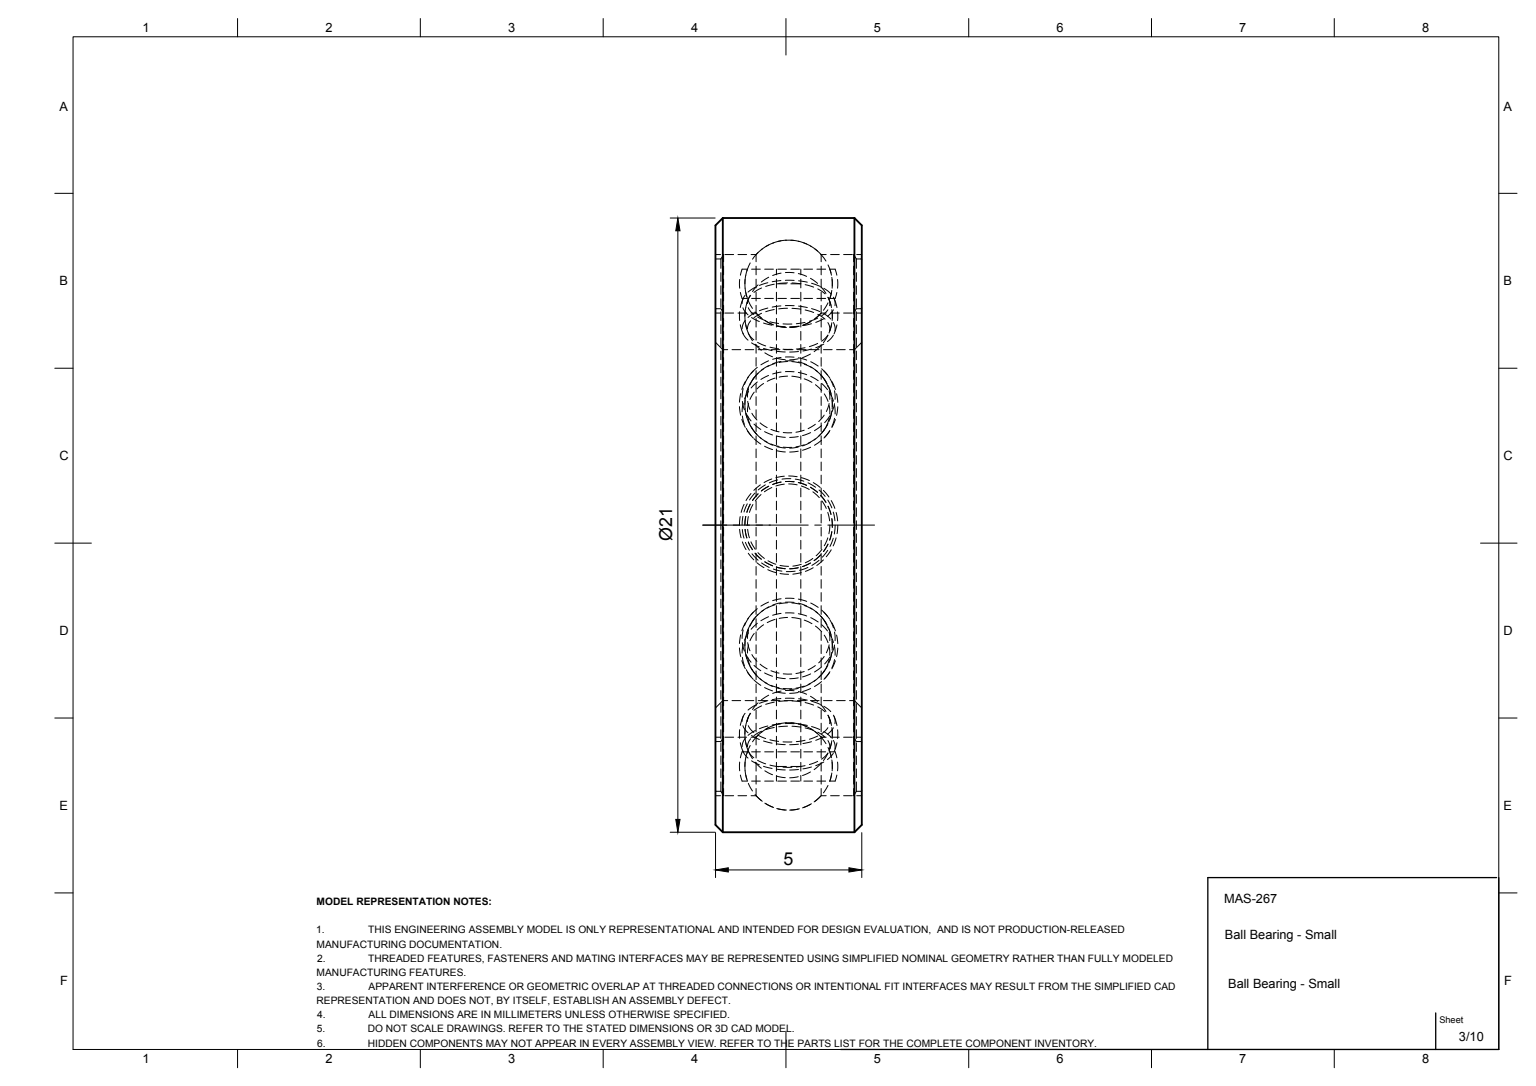
ISO-10303-21;
HEADER;
/* Generated by software containing ST-Developer
 * from STEP Tools, Inc. (www.steptools.com) 
 */

FILE_DESCRIPTION(
/* description */ (''),
/* implementation_level */ '2;1');

FILE_NAME(
/* name */ 'Ball Bearing - Small.step',
/* time_stamp */ '2026-10-12T15:29:24-07:00',
/* author */ (''),
/* organization */ (''),
/* preprocessor_version */ 'ST-DEVELOPER v20.2',
/* originating_system */ 'Autodesk Translation Framework v15.15.0.0',
/* authorisation */ '');

FILE_SCHEMA (('AUTOMOTIVE_DESIGN { 1 0 10303 214 3 1 1 }'));
ENDSEC;

DATA;
#10=MECHANICAL_DESIGN_GEOMETRIC_PRESENTATION_REPRESENTATION('',(#165,#166,#167,#168,#169,#170,#171,#172,#173,#174,#175,#176,#177,#178,#179,#180,#181,#182,#183,#184,#185,#186,#187,#188,#189,#190,#191,#192,#193),#9496);
#95=(
BOUNDED_SURFACE()
B_SPLINE_SURFACE(2,2,((#7928,#7929,#7930,#7931,#7932,#7933,#7934,#7935,
#7936),(#7937,#7938,#7939,#7940,#7941,#7942,#7943,#7944,#7945),(#7946,#7947,
#7948,#7949,#7950,#7951,#7952,#7953,#7954)),.UNSPECIFIED.,.F.,.T.,.F.)
B_SPLINE_SURFACE_WITH_KNOTS((3,3),(3,2,2,2,3),(-0.359817990374321,0.359817990374321),
(-3.14159265358979,-1.5707963267949,0.,1.5707963267949,3.14159265358979),
 .UNSPECIFIED.)
GEOMETRIC_REPRESENTATION_ITEM()
RATIONAL_B_SPLINE_SURFACE(((1.,0.707106781186548,1.,0.707106781186548,1.,
0.707106781186548,1.,0.707106781186548,1.),(0.935960925476955,0.661824317330392,
0.935960925476955,0.661824317330392,0.935960925476955,0.661824317330392,
0.935960925476955,0.661824317330392,0.935960925476955),(1.,0.707106781186548,
1.,0.707106781186548,1.,0.707106781186548,1.,0.707106781186548,1.)))
REPRESENTATION_ITEM('')
SURFACE()
);
#96=(
BOUNDED_SURFACE()
B_SPLINE_SURFACE(2,2,((#7970,#7971,#7972,#7973,#7974,#7975,#7976,#7977,
#7978),(#7979,#7980,#7981,#7982,#7983,#7984,#7985,#7986,#7987),(#7988,#7989,
#7990,#7991,#7992,#7993,#7994,#7995,#7996)),.UNSPECIFIED.,.F.,.T.,.F.)
B_SPLINE_SURFACE_WITH_KNOTS((3,3),(3,2,2,2,3),(-0.359817990374415,0.359817990374426),
(-3.14159265358979,-1.5707963267949,0.,1.5707963267949,3.14159265358979),
 .UNSPECIFIED.)
GEOMETRIC_REPRESENTATION_ITEM()
RATIONAL_B_SPLINE_SURFACE(((1.,0.707106781186548,1.,0.707106781186548,1.,
0.707106781186548,1.,0.707106781186548,1.),(0.935960925476919,0.661824317330366,
0.935960925476919,0.661824317330366,0.935960925476919,0.661824317330366,
0.935960925476919,0.661824317330366,0.935960925476919),(1.,0.707106781186548,
1.,0.707106781186548,1.,0.707106781186548,1.,0.707106781186548,1.)))
REPRESENTATION_ITEM('')
SURFACE()
);
#97=(
BOUNDED_SURFACE()
B_SPLINE_SURFACE(2,2,((#8012,#8013,#8014,#8015,#8016,#8017,#8018,#8019,
#8020),(#8021,#8022,#8023,#8024,#8025,#8026,#8027,#8028,#8029),(#8030,#8031,
#8032,#8033,#8034,#8035,#8036,#8037,#8038)),.UNSPECIFIED.,.F.,.T.,.F.)
B_SPLINE_SURFACE_WITH_KNOTS((3,3),(3,2,2,2,3),(-0.359817990374342,0.359817990374333),
(-3.14159265358979,-1.5707963267949,0.,1.5707963267949,3.14159265358979),
 .UNSPECIFIED.)
GEOMETRIC_REPRESENTATION_ITEM()
RATIONAL_B_SPLINE_SURFACE(((1.,0.707106781186548,1.,0.707106781186548,1.,
0.707106781186548,1.,0.707106781186548,1.),(0.935960925476941,0.661824317330382,
0.935960925476941,0.661824317330382,0.935960925476941,0.661824317330382,
0.935960925476941,0.661824317330382,0.935960925476941),(1.,0.707106781186548,
1.,0.707106781186548,1.,0.707106781186548,1.,0.707106781186548,1.)))
REPRESENTATION_ITEM('')
SURFACE()
);
#98=(
BOUNDED_SURFACE()
B_SPLINE_SURFACE(2,2,((#8054,#8055,#8056,#8057,#8058,#8059,#8060,#8061,
#8062),(#8063,#8064,#8065,#8066,#8067,#8068,#8069,#8070,#8071),(#8072,#8073,
#8074,#8075,#8076,#8077,#8078,#8079,#8080)),.UNSPECIFIED.,.F.,.T.,.F.)
B_SPLINE_SURFACE_WITH_KNOTS((3,3),(3,2,2,2,3),(-0.359817990374327,0.359817990374343),
(-3.14159265358979,-1.5707963267949,0.,1.5707963267949,3.14159265358979),
 .UNSPECIFIED.)
GEOMETRIC_REPRESENTATION_ITEM()
RATIONAL_B_SPLINE_SURFACE(((1.,0.707106781186548,1.,0.707106781186548,1.,
0.707106781186548,1.,0.707106781186548,1.),(0.935960925476945,0.661824317330385,
0.935960925476945,0.661824317330385,0.935960925476945,0.661824317330385,
0.935960925476945,0.661824317330385,0.935960925476945),(1.,0.707106781186548,
1.,0.707106781186548,1.,0.707106781186548,1.,0.707106781186548,1.)))
REPRESENTATION_ITEM('')
SURFACE()
);
#99=(
BOUNDED_SURFACE()
B_SPLINE_SURFACE(2,2,((#8096,#8097,#8098,#8099,#8100,#8101,#8102,#8103,
#8104),(#8105,#8106,#8107,#8108,#8109,#8110,#8111,#8112,#8113),(#8114,#8115,
#8116,#8117,#8118,#8119,#8120,#8121,#8122)),.UNSPECIFIED.,.F.,.T.,.F.)
B_SPLINE_SURFACE_WITH_KNOTS((3,3),(3,2,2,2,3),(-0.359817990374369,0.359817990374379),
(-3.14159265358979,-1.5707963267949,0.,1.5707963267949,3.14159265358979),
 .UNSPECIFIED.)
GEOMETRIC_REPRESENTATION_ITEM()
RATIONAL_B_SPLINE_SURFACE(((1.,0.707106781186548,1.,0.707106781186548,1.,
0.707106781186548,1.,0.707106781186548,1.),(0.935960925476939,0.661824317330381,
0.935960925476939,0.661824317330381,0.935960925476939,0.661824317330381,
0.935960925476939,0.661824317330381,0.935960925476939),(1.,0.707106781186548,
1.,0.707106781186548,1.,0.707106781186548,1.,0.707106781186548,1.)))
REPRESENTATION_ITEM('')
SURFACE()
);
#100=(
BOUNDED_SURFACE()
B_SPLINE_SURFACE(2,2,((#8138,#8139,#8140,#8141,#8142,#8143,#8144,#8145,
#8146),(#8147,#8148,#8149,#8150,#8151,#8152,#8153,#8154,#8155),(#8156,#8157,
#8158,#8159,#8160,#8161,#8162,#8163,#8164)),.UNSPECIFIED.,.F.,.T.,.F.)
B_SPLINE_SURFACE_WITH_KNOTS((3,3),(3,2,2,2,3),(-0.359817990374391,0.359817990374391),
(-3.14159265358979,-1.5707963267949,0.,1.5707963267949,3.14159265358979),
 .UNSPECIFIED.)
GEOMETRIC_REPRESENTATION_ITEM()
RATIONAL_B_SPLINE_SURFACE(((1.,0.707106781186548,1.,0.707106781186548,1.,
0.707106781186548,1.,0.707106781186548,1.),(0.935960925476929,0.661824317330373,
0.935960925476929,0.661824317330373,0.935960925476929,0.661824317330373,
0.935960925476929,0.661824317330373,0.935960925476929),(1.,0.707106781186548,
1.,0.707106781186548,1.,0.707106781186548,1.,0.707106781186548,1.)))
REPRESENTATION_ITEM('')
SURFACE()
);
#101=(
BOUNDED_SURFACE()
B_SPLINE_SURFACE(2,2,((#8180,#8181,#8182,#8183,#8184,#8185,#8186,#8187,
#8188),(#8189,#8190,#8191,#8192,#8193,#8194,#8195,#8196,#8197),(#8198,#8199,
#8200,#8201,#8202,#8203,#8204,#8205,#8206)),.UNSPECIFIED.,.F.,.T.,.F.)
B_SPLINE_SURFACE_WITH_KNOTS((3,3),(3,2,2,2,3),(-0.359817990374328,0.359817990374325),
(-3.14159265358979,-1.5707963267949,0.,1.5707963267949,3.14159265358979),
 .UNSPECIFIED.)
GEOMETRIC_REPRESENTATION_ITEM()
RATIONAL_B_SPLINE_SURFACE(((1.,0.707106781186548,1.,0.707106781186548,1.,
0.707106781186548,1.,0.707106781186548,1.),(0.935960925476951,0.661824317330389,
0.935960925476951,0.661824317330389,0.935960925476951,0.661824317330389,
0.935960925476951,0.661824317330389,0.935960925476951),(1.,0.707106781186548,
1.,0.707106781186548,1.,0.707106781186548,1.,0.707106781186548,1.)))
REPRESENTATION_ITEM('')
SURFACE()
);
#102=(
BOUNDED_SURFACE()
B_SPLINE_SURFACE(2,2,((#8222,#8223,#8224,#8225,#8226,#8227,#8228,#8229,
#8230),(#8231,#8232,#8233,#8234,#8235,#8236,#8237,#8238,#8239),(#8240,#8241,
#8242,#8243,#8244,#8245,#8246,#8247,#8248)),.UNSPECIFIED.,.F.,.T.,.F.)
B_SPLINE_SURFACE_WITH_KNOTS((3,3),(3,2,2,2,3),(-0.359817990374346,0.359817990374343),
(-3.14159265358979,-1.5707963267949,0.,1.5707963267949,3.14159265358979),
 .UNSPECIFIED.)
GEOMETRIC_REPRESENTATION_ITEM()
RATIONAL_B_SPLINE_SURFACE(((1.,0.707106781186548,1.,0.707106781186548,1.,
0.707106781186548,1.,0.707106781186548,1.),(0.935960925476942,0.661824317330383,
0.935960925476942,0.661824317330383,0.935960925476942,0.661824317330383,
0.935960925476942,0.661824317330383,0.935960925476942),(1.,0.707106781186548,
1.,0.707106781186548,1.,0.707106781186548,1.,0.707106781186548,1.)))
REPRESENTATION_ITEM('')
SURFACE()
);
#103=(
BOUNDED_SURFACE()
B_SPLINE_SURFACE(2,2,((#8264,#8265,#8266,#8267,#8268,#8269,#8270,#8271,
#8272),(#8273,#8274,#8275,#8276,#8277,#8278,#8279,#8280,#8281),(#8282,#8283,
#8284,#8285,#8286,#8287,#8288,#8289,#8290)),.UNSPECIFIED.,.F.,.T.,.F.)
B_SPLINE_SURFACE_WITH_KNOTS((3,3),(3,2,2,2,3),(-0.359817990374353,0.359817990374347),
(-3.14159265358979,-1.5707963267949,0.,1.5707963267949,3.14159265358979),
 .UNSPECIFIED.)
GEOMETRIC_REPRESENTATION_ITEM()
RATIONAL_B_SPLINE_SURFACE(((1.,0.707106781186548,1.,0.707106781186548,1.,
0.707106781186548,1.,0.707106781186548,1.),(0.935960925476944,0.661824317330384,
0.935960925476944,0.661824317330384,0.935960925476944,0.661824317330384,
0.935960925476944,0.661824317330384,0.935960925476944),(1.,0.707106781186548,
1.,0.707106781186548,1.,0.707106781186548,1.,0.707106781186548,1.)))
REPRESENTATION_ITEM('')
SURFACE()
);
#104=(
BOUNDED_SURFACE()
B_SPLINE_SURFACE(2,2,((#8306,#8307,#8308,#8309,#8310,#8311,#8312,#8313,
#8314),(#8315,#8316,#8317,#8318,#8319,#8320,#8321,#8322,#8323),(#8324,#8325,
#8326,#8327,#8328,#8329,#8330,#8331,#8332)),.UNSPECIFIED.,.F.,.T.,.F.)
B_SPLINE_SURFACE_WITH_KNOTS((3,3),(3,2,2,2,3),(-0.359817990374389,0.359817990374389),
(-3.14159265358979,-1.5707963267949,0.,1.5707963267949,3.14159265358979),
 .UNSPECIFIED.)
GEOMETRIC_REPRESENTATION_ITEM()
RATIONAL_B_SPLINE_SURFACE(((1.,0.707106781186548,1.,0.707106781186548,1.,
0.707106781186548,1.,0.707106781186548,1.),(0.935960925476925,0.661824317330371,
0.935960925476925,0.661824317330371,0.935960925476925,0.661824317330371,
0.935960925476925,0.661824317330371,0.935960925476925),(1.,0.707106781186548,
1.,0.707106781186548,1.,0.707106781186548,1.,0.707106781186548,1.)))
REPRESENTATION_ITEM('')
SURFACE()
);
#105=(
BOUNDED_SURFACE()
B_SPLINE_SURFACE(2,2,((#8362,#8363,#8364,#8365,#8366,#8367,#8368,#8369,
#8370),(#8371,#8372,#8373,#8374,#8375,#8376,#8377,#8378,#8379),(#8380,#8381,
#8382,#8383,#8384,#8385,#8386,#8387,#8388)),.UNSPECIFIED.,.F.,.T.,.F.)
B_SPLINE_SURFACE_WITH_KNOTS((3,3),(3,2,2,2,3),(-0.359817990374337,0.359817990374338),
(-3.14159265358979,-1.5707963267949,0.,1.5707963267949,3.14159265358979),
 .UNSPECIFIED.)
GEOMETRIC_REPRESENTATION_ITEM()
RATIONAL_B_SPLINE_SURFACE(((1.,0.707106781186548,1.,0.707106781186548,1.,
0.707106781186548,1.,0.707106781186548,1.),(0.935960925476947,0.661824317330386,
0.935960925476947,0.661824317330386,0.935960925476947,0.661824317330386,
0.935960925476947,0.661824317330386,0.935960925476947),(1.,0.707106781186548,
1.,0.707106781186548,1.,0.707106781186548,1.,0.707106781186548,1.)))
REPRESENTATION_ITEM('')
SURFACE()
);
#106=(
BOUNDED_SURFACE()
B_SPLINE_SURFACE(2,2,((#8404,#8405,#8406,#8407,#8408,#8409,#8410,#8411,
#8412),(#8413,#8414,#8415,#8416,#8417,#8418,#8419,#8420,#8421),(#8422,#8423,
#8424,#8425,#8426,#8427,#8428,#8429,#8430)),.UNSPECIFIED.,.F.,.T.,.F.)
B_SPLINE_SURFACE_WITH_KNOTS((3,3),(3,2,2,2,3),(-0.359817990374313,0.359817990374317),
(-3.14159265358979,-1.5707963267949,0.,1.5707963267949,3.14159265358979),
 .UNSPECIFIED.)
GEOMETRIC_REPRESENTATION_ITEM()
RATIONAL_B_SPLINE_SURFACE(((1.,0.707106781186548,1.,0.707106781186548,1.,
0.707106781186548,1.,0.707106781186548,1.),(0.935960925476952,0.66182431733039,
0.935960925476952,0.66182431733039,0.935960925476952,0.66182431733039,0.935960925476952,
0.66182431733039,0.935960925476952),(1.,0.707106781186548,1.,0.707106781186548,
1.,0.707106781186548,1.,0.707106781186548,1.)))
REPRESENTATION_ITEM('')
SURFACE()
);
#107=CONICAL_SURFACE('',#5303,6.24999999999999,0.785398163397428);
#108=CONICAL_SURFACE('',#5309,6.,0.785398163397428);
#109=CONICAL_SURFACE('',#5319,10.25,0.785398163397433);
#110=CONICAL_SURFACE('',#5330,10.5,0.785398163397433);
#111=CONICAL_SURFACE('',#5488,9.25000000000001,1.01776488264426);
#112=CONICAL_SURFACE('',#5490,7.39999999999999,1.01776488264426);
#113=CONICAL_SURFACE('',#5507,7.24999999999999,1.01776488264426);
#114=CONICAL_SURFACE('',#5509,9.1,1.01776488264426);
#124=TOROIDAL_SURFACE('',#5299,8.25,1.49484711634153);
#125=TOROIDAL_SURFACE('',#5325,8.25,1.49484711634153);
#126=TOROIDAL_SURFACE('',#5475,7.42777777777777,0.0277777777777778);
#127=TOROIDAL_SURFACE('',#5480,9.07222222222223,0.0277777777777778);
#128=TOROIDAL_SURFACE('',#5496,9.07222222222222,0.027777777777778);
#129=TOROIDAL_SURFACE('',#5500,7.42777777777777,0.027777777777778);
#147=SHAPE_REPRESENTATION_RELATIONSHIP('SRR','None',#9541,#156);
#156=ADVANCED_BREP_SHAPE_REPRESENTATION('',(#222,#223,#224,#225,#226,#227,
#228,#229,#230,#231,#232,#233,#234,#235,#236,#237,#238,#239,#240,#241,#242,
#243,#244,#245,#246,#247,#248,#249,#250),#9489);
#165=STYLED_ITEM('',(#9594),#222);
#166=STYLED_ITEM('',(#9594),#223);
#167=STYLED_ITEM('',(#9594),#224);
#168=STYLED_ITEM('',(#9594),#225);
#169=STYLED_ITEM('',(#9594),#226);
#170=STYLED_ITEM('',(#9594),#227);
#171=STYLED_ITEM('',(#9594),#228);
#172=STYLED_ITEM('',(#9594),#229);
#173=STYLED_ITEM('',(#9594),#230);
#174=STYLED_ITEM('',(#9594),#231);
#175=STYLED_ITEM('',(#9594),#232);
#176=STYLED_ITEM('',(#9594),#233);
#177=STYLED_ITEM('',(#9594),#234);
#178=STYLED_ITEM('',(#9594),#235);
#179=STYLED_ITEM('',(#9594),#236);
#180=STYLED_ITEM('',(#9594),#237);
#181=STYLED_ITEM('',(#9594),#238);
#182=STYLED_ITEM('',(#9594),#239);
#183=STYLED_ITEM('',(#9594),#240);
#184=STYLED_ITEM('',(#9594),#241);
#185=STYLED_ITEM('',(#9594),#242);
#186=STYLED_ITEM('',(#9594),#243);
#187=STYLED_ITEM('',(#9594),#244);
#188=STYLED_ITEM('',(#9594),#245);
#189=STYLED_ITEM('',(#9594),#246);
#190=STYLED_ITEM('',(#9594),#247);
#191=STYLED_ITEM('',(#9594),#248);
#192=STYLED_ITEM('',(#9594),#249);
#193=STYLED_ITEM('',(#9594),#250);
#222=MANIFOLD_SOLID_BREP('Body1',#4967);
#223=MANIFOLD_SOLID_BREP('Body2',#4968);
#224=MANIFOLD_SOLID_BREP('Body3',#4969);
#225=MANIFOLD_SOLID_BREP('Body4',#4970);
#226=MANIFOLD_SOLID_BREP('Body5',#4971);
#227=MANIFOLD_SOLID_BREP('Body6',#4972);
#228=MANIFOLD_SOLID_BREP('Body7',#4973);
#229=MANIFOLD_SOLID_BREP('Body8',#4974);
#230=MANIFOLD_SOLID_BREP('Body9',#4975);
#231=MANIFOLD_SOLID_BREP('Body10',#4976);
#232=MANIFOLD_SOLID_BREP('Body11',#4977);
#233=MANIFOLD_SOLID_BREP('Body12',#4978);
#234=MANIFOLD_SOLID_BREP('Body13',#4979);
#235=MANIFOLD_SOLID_BREP('Body14',#4980);
#236=MANIFOLD_SOLID_BREP('Body15',#4981);
#237=MANIFOLD_SOLID_BREP('Body16',#4982);
#238=MANIFOLD_SOLID_BREP('Body17',#4983);
#239=MANIFOLD_SOLID_BREP('Body18',#4984);
#240=MANIFOLD_SOLID_BREP('Body19',#4985);
#241=MANIFOLD_SOLID_BREP('Body20',#4986);
#242=MANIFOLD_SOLID_BREP('Body21',#4987);
#243=MANIFOLD_SOLID_BREP('Body22',#4988);
#244=MANIFOLD_SOLID_BREP('Body23',#4989);
#245=MANIFOLD_SOLID_BREP('Body24',#4990);
#246=MANIFOLD_SOLID_BREP('Body25',#4991);
#247=MANIFOLD_SOLID_BREP('Body26',#4992);
#248=MANIFOLD_SOLID_BREP('Body27',#4993);
#249=MANIFOLD_SOLID_BREP('Body28',#4994);
#250=MANIFOLD_SOLID_BREP('Body29',#4995);
#293=SPHERICAL_SURFACE('',#5317,1.49484711634153);
#294=SPHERICAL_SURFACE('',#5337,1.49484711634153);
#295=SPHERICAL_SURFACE('',#5339,1.49484711634153);
#296=SPHERICAL_SURFACE('',#5341,1.49484711634153);
#297=SPHERICAL_SURFACE('',#5343,1.49484711634153);
#298=SPHERICAL_SURFACE('',#5345,1.49484711634153);
#299=SPHERICAL_SURFACE('',#5347,1.49484711634153);
#300=SPHERICAL_SURFACE('',#5349,1.49484711634153);
#301=SPHERICAL_SURFACE('',#5351,1.49484711634153);
#302=SPHERICAL_SURFACE('',#5353,1.49484711634153);
#303=SPHERICAL_SURFACE('',#5358,1.49484711634152);
#304=SPHERICAL_SURFACE('',#5367,1.49484711634152);
#305=SPHERICAL_SURFACE('',#5376,1.49484711634152);
#306=SPHERICAL_SURFACE('',#5385,1.49484711634152);
#307=SPHERICAL_SURFACE('',#5394,1.49484711634152);
#308=SPHERICAL_SURFACE('',#5403,1.49484711634152);
#309=SPHERICAL_SURFACE('',#5412,1.49484711634152);
#310=SPHERICAL_SURFACE('',#5421,1.49484711634152);
#311=SPHERICAL_SURFACE('',#5430,1.49484711634152);
#312=SPHERICAL_SURFACE('',#5439,1.49484711634152);
#313=SPHERICAL_SURFACE('',#5456,1.49484711634152);
#314=SPHERICAL_SURFACE('',#5465,1.49484711634152);
#315=SPHERICAL_SURFACE('',#5471,1.49484711634153);
#316=SPHERICAL_SURFACE('',#5473,1.49484711634153);
#354=FACE_BOUND('',#1069,.T.);
#355=FACE_BOUND('',#1071,.T.);
#356=FACE_BOUND('',#1080,.T.);
#357=FACE_BOUND('',#1082,.T.);
#358=FACE_BOUND('',#1094,.T.);
#359=FACE_BOUND('',#1095,.T.);
#360=FACE_BOUND('',#1097,.T.);
#361=FACE_BOUND('',#1099,.T.);
#362=FACE_BOUND('',#1102,.T.);
#363=FACE_BOUND('',#1103,.T.);
#364=FACE_BOUND('',#1105,.T.);
#365=FACE_BOUND('',#1107,.T.);
#366=FACE_BOUND('',#1110,.T.);
#367=FACE_BOUND('',#1111,.T.);
#368=FACE_BOUND('',#1113,.T.);
#369=FACE_BOUND('',#1115,.T.);
#370=FACE_BOUND('',#1118,.T.);
#371=FACE_BOUND('',#1119,.T.);
#372=FACE_BOUND('',#1121,.T.);
#373=FACE_BOUND('',#1123,.T.);
#374=FACE_BOUND('',#1126,.T.);
#375=FACE_BOUND('',#1127,.T.);
#376=FACE_BOUND('',#1129,.T.);
#377=FACE_BOUND('',#1131,.T.);
#378=FACE_BOUND('',#1134,.T.);
#379=FACE_BOUND('',#1135,.T.);
#380=FACE_BOUND('',#1137,.T.);
#381=FACE_BOUND('',#1139,.T.);
#382=FACE_BOUND('',#1142,.T.);
#383=FACE_BOUND('',#1143,.T.);
#384=FACE_BOUND('',#1145,.T.);
#385=FACE_BOUND('',#1147,.T.);
#386=FACE_BOUND('',#1150,.T.);
#387=FACE_BOUND('',#1151,.T.);
#388=FACE_BOUND('',#1153,.T.);
#389=FACE_BOUND('',#1155,.T.);
#390=FACE_BOUND('',#1158,.T.);
#391=FACE_BOUND('',#1159,.T.);
#392=FACE_BOUND('',#1161,.T.);
#393=FACE_BOUND('',#1163,.T.);
#394=FACE_BOUND('',#1166,.T.);
#395=FACE_BOUND('',#1167,.T.);
#396=FACE_BOUND('',#1169,.T.);
#397=FACE_BOUND('',#1171,.T.);
#398=FACE_BOUND('',#1175,.T.);
#399=FACE_BOUND('',#1177,.T.);
#400=FACE_BOUND('',#1180,.T.);
#401=FACE_BOUND('',#1181,.T.);
#402=FACE_BOUND('',#1183,.T.);
#403=FACE_BOUND('',#1185,.T.);
#404=FACE_BOUND('',#1188,.T.);
#405=FACE_BOUND('',#1189,.T.);
#406=FACE_BOUND('',#1191,.T.);
#407=FACE_BOUND('',#1193,.T.);
#408=FACE_BOUND('',#1203,.T.);
#409=FACE_BOUND('',#1205,.T.);
#410=FACE_BOUND('',#1213,.T.);
#411=FACE_BOUND('',#1215,.T.);
#511=PLANE('',#5315);
#512=PLANE('',#5316);
#513=PLANE('',#5335);
#514=PLANE('',#5336);
#515=PLANE('',#5362);
#516=PLANE('',#5363);
#517=PLANE('',#5371);
#518=PLANE('',#5372);
#519=PLANE('',#5380);
#520=PLANE('',#5381);
#521=PLANE('',#5389);
#522=PLANE('',#5390);
#523=PLANE('',#5398);
#524=PLANE('',#5399);
#525=PLANE('',#5407);
#526=PLANE('',#5408);
#527=PLANE('',#5416);
#528=PLANE('',#5417);
#529=PLANE('',#5425);
#530=PLANE('',#5426);
#531=PLANE('',#5434);
#532=PLANE('',#5435);
#533=PLANE('',#5443);
#534=PLANE('',#5444);
#535=PLANE('',#5451);
#536=PLANE('',#5452);
#537=PLANE('',#5460);
#538=PLANE('',#5461);
#539=PLANE('',#5469);
#540=PLANE('',#5470);
#541=PLANE('',#5494);
#542=PLANE('',#5495);
#543=PLANE('',#5513);
#544=PLANE('',#5514);
#709=FACE_OUTER_BOUND('',#1062,.T.);
#710=FACE_OUTER_BOUND('',#1063,.T.);
#711=FACE_OUTER_BOUND('',#1064,.T.);
#712=FACE_OUTER_BOUND('',#1065,.T.);
#713=FACE_OUTER_BOUND('',#1066,.T.);
#714=FACE_OUTER_BOUND('',#1067,.T.);
#715=FACE_OUTER_BOUND('',#1068,.T.);
#716=FACE_OUTER_BOUND('',#1070,.T.);
#717=FACE_OUTER_BOUND('',#1072,.T.);
#718=FACE_OUTER_BOUND('',#1073,.T.);
#719=FACE_OUTER_BOUND('',#1074,.T.);
#720=FACE_OUTER_BOUND('',#1075,.T.);
#721=FACE_OUTER_BOUND('',#1076,.T.);
#722=FACE_OUTER_BOUND('',#1077,.T.);
#723=FACE_OUTER_BOUND('',#1078,.T.);
#724=FACE_OUTER_BOUND('',#1079,.T.);
#725=FACE_OUTER_BOUND('',#1081,.T.);
#726=FACE_OUTER_BOUND('',#1083,.T.);
#727=FACE_OUTER_BOUND('',#1084,.T.);
#728=FACE_OUTER_BOUND('',#1085,.T.);
#729=FACE_OUTER_BOUND('',#1086,.T.);
#730=FACE_OUTER_BOUND('',#1087,.T.);
#731=FACE_OUTER_BOUND('',#1088,.T.);
#732=FACE_OUTER_BOUND('',#1089,.T.);
#733=FACE_OUTER_BOUND('',#1090,.T.);
#734=FACE_OUTER_BOUND('',#1091,.T.);
#735=FACE_OUTER_BOUND('',#1092,.T.);
#736=FACE_OUTER_BOUND('',#1093,.T.);
#737=FACE_OUTER_BOUND('',#1096,.T.);
#738=FACE_OUTER_BOUND('',#1098,.T.);
#739=FACE_OUTER_BOUND('',#1100,.T.);
#740=FACE_OUTER_BOUND('',#1101,.T.);
#741=FACE_OUTER_BOUND('',#1104,.T.);
#742=FACE_OUTER_BOUND('',#1106,.T.);
#743=FACE_OUTER_BOUND('',#1108,.T.);
#744=FACE_OUTER_BOUND('',#1109,.T.);
#745=FACE_OUTER_BOUND('',#1112,.T.);
#746=FACE_OUTER_BOUND('',#1114,.T.);
#747=FACE_OUTER_BOUND('',#1116,.T.);
#748=FACE_OUTER_BOUND('',#1117,.T.);
#749=FACE_OUTER_BOUND('',#1120,.T.);
#750=FACE_OUTER_BOUND('',#1122,.T.);
#751=FACE_OUTER_BOUND('',#1124,.T.);
#752=FACE_OUTER_BOUND('',#1125,.T.);
#753=FACE_OUTER_BOUND('',#1128,.T.);
#754=FACE_OUTER_BOUND('',#1130,.T.);
#755=FACE_OUTER_BOUND('',#1132,.T.);
#756=FACE_OUTER_BOUND('',#1133,.T.);
#757=FACE_OUTER_BOUND('',#1136,.T.);
#758=FACE_OUTER_BOUND('',#1138,.T.);
#759=FACE_OUTER_BOUND('',#1140,.T.);
#760=FACE_OUTER_BOUND('',#1141,.T.);
#761=FACE_OUTER_BOUND('',#1144,.T.);
#762=FACE_OUTER_BOUND('',#1146,.T.);
#763=FACE_OUTER_BOUND('',#1148,.T.);
#764=FACE_OUTER_BOUND('',#1149,.T.);
#765=FACE_OUTER_BOUND('',#1152,.T.);
#766=FACE_OUTER_BOUND('',#1154,.T.);
#767=FACE_OUTER_BOUND('',#1156,.T.);
#768=FACE_OUTER_BOUND('',#1157,.T.);
#769=FACE_OUTER_BOUND('',#1160,.T.);
#770=FACE_OUTER_BOUND('',#1162,.T.);
#771=FACE_OUTER_BOUND('',#1164,.T.);
#772=FACE_OUTER_BOUND('',#1165,.T.);
#773=FACE_OUTER_BOUND('',#1168,.T.);
#774=FACE_OUTER_BOUND('',#1170,.T.);
#775=FACE_OUTER_BOUND('',#1172,.T.);
#776=FACE_OUTER_BOUND('',#1173,.T.);
#777=FACE_OUTER_BOUND('',#1174,.T.);
#778=FACE_OUTER_BOUND('',#1176,.T.);
#779=FACE_OUTER_BOUND('',#1178,.T.);
#780=FACE_OUTER_BOUND('',#1179,.T.);
#781=FACE_OUTER_BOUND('',#1182,.T.);
#782=FACE_OUTER_BOUND('',#1184,.T.);
#783=FACE_OUTER_BOUND('',#1186,.T.);
#784=FACE_OUTER_BOUND('',#1187,.T.);
#785=FACE_OUTER_BOUND('',#1190,.T.);
#786=FACE_OUTER_BOUND('',#1192,.T.);
#787=FACE_OUTER_BOUND('',#1194,.T.);
#788=FACE_OUTER_BOUND('',#1195,.T.);
#789=FACE_OUTER_BOUND('',#1196,.T.);
#790=FACE_OUTER_BOUND('',#1197,.T.);
#791=FACE_OUTER_BOUND('',#1198,.T.);
#792=FACE_OUTER_BOUND('',#1199,.T.);
#793=FACE_OUTER_BOUND('',#1200,.T.);
#794=FACE_OUTER_BOUND('',#1201,.T.);
#795=FACE_OUTER_BOUND('',#1202,.T.);
#796=FACE_OUTER_BOUND('',#1204,.T.);
#797=FACE_OUTER_BOUND('',#1206,.T.);
#798=FACE_OUTER_BOUND('',#1207,.T.);
#799=FACE_OUTER_BOUND('',#1208,.T.);
#800=FACE_OUTER_BOUND('',#1209,.T.);
#801=FACE_OUTER_BOUND('',#1210,.T.);
#802=FACE_OUTER_BOUND('',#1211,.T.);
#803=FACE_OUTER_BOUND('',#1212,.T.);
#804=FACE_OUTER_BOUND('',#1214,.T.);
#1062=EDGE_LOOP('',(#3657,#3658,#3659,#3660));
#1063=EDGE_LOOP('',(#3661,#3662,#3663,#3664));
#1064=EDGE_LOOP('',(#3665,#3666,#3667,#3668,#3669));
#1065=EDGE_LOOP('',(#3670,#3671,#3672,#3673,#3674));
#1066=EDGE_LOOP('',(#3675,#3676,#3677,#3678));
#1067=EDGE_LOOP('',(#3679,#3680,#3681,#3682));
#1068=EDGE_LOOP('',(#3683));
#1069=EDGE_LOOP('',(#3684));
#1070=EDGE_LOOP('',(#3685));
#1071=EDGE_LOOP('',(#3686));
#1072=EDGE_LOOP('',(#3687,#3688));
#1073=EDGE_LOOP('',(#3689,#3690,#3691,#3692));
#1074=EDGE_LOOP('',(#3693,#3694,#3695,#3696));
#1075=EDGE_LOOP('',(#3697,#3698,#3699,#3700));
#1076=EDGE_LOOP('',(#3701,#3702,#3703,#3704));
#1077=EDGE_LOOP('',(#3705,#3706,#3707,#3708,#3709));
#1078=EDGE_LOOP('',(#3710,#3711,#3712,#3713,#3714));
#1079=EDGE_LOOP('',(#3715));
#1080=EDGE_LOOP('',(#3716));
#1081=EDGE_LOOP('',(#3717));
#1082=EDGE_LOOP('',(#3718));
#1083=EDGE_LOOP('',(#3719,#3720));
#1084=EDGE_LOOP('',(#3721,#3722));
#1085=EDGE_LOOP('',(#3723,#3724));
#1086=EDGE_LOOP('',(#3725,#3726));
#1087=EDGE_LOOP('',(#3727,#3728));
#1088=EDGE_LOOP('',(#3729,#3730));
#1089=EDGE_LOOP('',(#3731,#3732));
#1090=EDGE_LOOP('',(#3733,#3734));
#1091=EDGE_LOOP('',(#3735,#3736));
#1092=EDGE_LOOP('',(#3737,#3738,#3739,#3740));
#1093=EDGE_LOOP('',(#3741,#3742));
#1094=EDGE_LOOP('',(#3743));
#1095=EDGE_LOOP('',(#3744));
#1096=EDGE_LOOP('',(#3745));
#1097=EDGE_LOOP('',(#3746));
#1098=EDGE_LOOP('',(#3747));
#1099=EDGE_LOOP('',(#3748));
#1100=EDGE_LOOP('',(#3749,#3750,#3751,#3752));
#1101=EDGE_LOOP('',(#3753,#3754));
#1102=EDGE_LOOP('',(#3755));
#1103=EDGE_LOOP('',(#3756));
#1104=EDGE_LOOP('',(#3757));
#1105=EDGE_LOOP('',(#3758));
#1106=EDGE_LOOP('',(#3759));
#1107=EDGE_LOOP('',(#3760));
#1108=EDGE_LOOP('',(#3761,#3762,#3763,#3764));
#1109=EDGE_LOOP('',(#3765,#3766));
#1110=EDGE_LOOP('',(#3767));
#1111=EDGE_LOOP('',(#3768));
#1112=EDGE_LOOP('',(#3769));
#1113=EDGE_LOOP('',(#3770));
#1114=EDGE_LOOP('',(#3771));
#1115=EDGE_LOOP('',(#3772));
#1116=EDGE_LOOP('',(#3773,#3774,#3775,#3776));
#1117=EDGE_LOOP('',(#3777,#3778));
#1118=EDGE_LOOP('',(#3779));
#1119=EDGE_LOOP('',(#3780));
#1120=EDGE_LOOP('',(#3781));
#1121=EDGE_LOOP('',(#3782));
#1122=EDGE_LOOP('',(#3783));
#1123=EDGE_LOOP('',(#3784));
#1124=EDGE_LOOP('',(#3785,#3786,#3787,#3788));
#1125=EDGE_LOOP('',(#3789,#3790));
#1126=EDGE_LOOP('',(#3791));
#1127=EDGE_LOOP('',(#3792));
#1128=EDGE_LOOP('',(#3793));
#1129=EDGE_LOOP('',(#3794));
#1130=EDGE_LOOP('',(#3795));
#1131=EDGE_LOOP('',(#3796));
#1132=EDGE_LOOP('',(#3797,#3798,#3799,#3800));
#1133=EDGE_LOOP('',(#3801,#3802));
#1134=EDGE_LOOP('',(#3803));
#1135=EDGE_LOOP('',(#3804));
#1136=EDGE_LOOP('',(#3805));
#1137=EDGE_LOOP('',(#3806));
#1138=EDGE_LOOP('',(#3807));
#1139=EDGE_LOOP('',(#3808));
#1140=EDGE_LOOP('',(#3809,#3810,#3811,#3812));
#1141=EDGE_LOOP('',(#3813,#3814));
#1142=EDGE_LOOP('',(#3815));
#1143=EDGE_LOOP('',(#3816));
#1144=EDGE_LOOP('',(#3817));
#1145=EDGE_LOOP('',(#3818));
#1146=EDGE_LOOP('',(#3819));
#1147=EDGE_LOOP('',(#3820));
#1148=EDGE_LOOP('',(#3821,#3822,#3823,#3824));
#1149=EDGE_LOOP('',(#3825,#3826));
#1150=EDGE_LOOP('',(#3827));
#1151=EDGE_LOOP('',(#3828));
#1152=EDGE_LOOP('',(#3829));
#1153=EDGE_LOOP('',(#3830));
#1154=EDGE_LOOP('',(#3831));
#1155=EDGE_LOOP('',(#3832));
#1156=EDGE_LOOP('',(#3833,#3834,#3835,#3836));
#1157=EDGE_LOOP('',(#3837,#3838));
#1158=EDGE_LOOP('',(#3839));
#1159=EDGE_LOOP('',(#3840));
#1160=EDGE_LOOP('',(#3841));
#1161=EDGE_LOOP('',(#3842));
#1162=EDGE_LOOP('',(#3843));
#1163=EDGE_LOOP('',(#3844));
#1164=EDGE_LOOP('',(#3845,#3846,#3847,#3848));
#1165=EDGE_LOOP('',(#3849,#3850));
#1166=EDGE_LOOP('',(#3851));
#1167=EDGE_LOOP('',(#3852));
#1168=EDGE_LOOP('',(#3853));
#1169=EDGE_LOOP('',(#3854));
#1170=EDGE_LOOP('',(#3855));
#1171=EDGE_LOOP('',(#3856));
#1172=EDGE_LOOP('',(#3857,#3858,#3859,#3860));
#1173=EDGE_LOOP('',(#3861,#3862,#3863,#3864));
#1174=EDGE_LOOP('',(#3865));
#1175=EDGE_LOOP('',(#3866));
#1176=EDGE_LOOP('',(#3867));
#1177=EDGE_LOOP('',(#3868));
#1178=EDGE_LOOP('',(#3869,#3870,#3871,#3872));
#1179=EDGE_LOOP('',(#3873,#3874));
#1180=EDGE_LOOP('',(#3875));
#1181=EDGE_LOOP('',(#3876));
#1182=EDGE_LOOP('',(#3877));
#1183=EDGE_LOOP('',(#3878));
#1184=EDGE_LOOP('',(#3879));
#1185=EDGE_LOOP('',(#3880));
#1186=EDGE_LOOP('',(#3881,#3882,#3883,#3884));
#1187=EDGE_LOOP('',(#3885,#3886));
#1188=EDGE_LOOP('',(#3887));
#1189=EDGE_LOOP('',(#3888));
#1190=EDGE_LOOP('',(#3889));
#1191=EDGE_LOOP('',(#3890));
#1192=EDGE_LOOP('',(#3891));
#1193=EDGE_LOOP('',(#3892));
#1194=EDGE_LOOP('',(#3893,#3894));
#1195=EDGE_LOOP('',(#3895,#3896));
#1196=EDGE_LOOP('',(#3897,#3898,#3899,#3900,#3901));
#1197=EDGE_LOOP('',(#3902,#3903,#3904,#3905,#3906));
#1198=EDGE_LOOP('',(#3907,#3908,#3909,#3910,#3911,#3912));
#1199=EDGE_LOOP('',(#3913,#3914,#3915,#3916,#3917));
#1200=EDGE_LOOP('',(#3918,#3919,#3920,#3921));
#1201=EDGE_LOOP('',(#3922,#3923,#3924,#3925,#3926));
#1202=EDGE_LOOP('',(#3927));
#1203=EDGE_LOOP('',(#3928));
#1204=EDGE_LOOP('',(#3929));
#1205=EDGE_LOOP('',(#3930));
#1206=EDGE_LOOP('',(#3931,#3932,#3933,#3934));
#1207=EDGE_LOOP('',(#3935,#3936,#3937,#3938));
#1208=EDGE_LOOP('',(#3939,#3940,#3941,#3942,#3943));
#1209=EDGE_LOOP('',(#3944,#3945,#3946,#3947,#3948));
#1210=EDGE_LOOP('',(#3949,#3950,#3951,#3952));
#1211=EDGE_LOOP('',(#3953,#3954,#3955,#3956));
#1212=EDGE_LOOP('',(#3957));
#1213=EDGE_LOOP('',(#3958));
#1214=EDGE_LOOP('',(#3959));
#1215=EDGE_LOOP('',(#3960));
#1515=LINE('',#7834,#1752);
#1516=LINE('',#7838,#1753);
#1517=LINE('',#7844,#1754);
#1518=LINE('',#7849,#1755);
#1519=LINE('',#7852,#1756);
#1520=LINE('',#7864,#1757);
#1521=LINE('',#7870,#1758);
#1522=LINE('',#7879,#1759);
#1523=LINE('',#7886,#1760);
#1524=LINE('',#7889,#1761);
#1525=LINE('',#8352,#1762);
#1526=LINE('',#8358,#1763);
#1527=LINE('',#8475,#1764);
#1528=LINE('',#8479,#1765);
#1529=LINE('',#8484,#1766);
#1530=LINE('',#8487,#1767);
#1531=LINE('',#8507,#1768);
#1532=LINE('',#8511,#1769);
#1533=LINE('',#8516,#1770);
#1534=LINE('',#8519,#1771);
#1752=VECTOR('',#6272,6.24999999999999);
#1753=VECTOR('',#6277,6.);
#1754=VECTOR('',#6284,6.);
#1755=VECTOR('',#6291,7.24999999999999);
#1756=VECTOR('',#6294,7.24999999999999);
#1757=VECTOR('',#6309,10.25);
#1758=VECTOR('',#6316,9.25000000000001);
#1759=VECTOR('',#6329,9.25);
#1760=VECTOR('',#6336,10.5);
#1761=VECTOR('',#6341,10.5);
#1762=VECTOR('',#6566,8.25);
#1763=VECTOR('',#6573,8.75);
#1764=VECTOR('',#6650,9.1);
#1765=VECTOR('',#6655,9.25000000000001);
#1766=VECTOR('',#6660,7.39999999999999);
#1767=VECTOR('',#6665,7.39999999999999);
#1768=VECTOR('',#6692,7.39999999999999);
#1769=VECTOR('',#6697,7.24999999999999);
#1770=VECTOR('',#6702,9.1);
#1771=VECTOR('',#6707,9.1);
#1993=CIRCLE('',#5300,7.24999999999999);
#1994=CIRCLE('',#5301,1.49484711634153);
#1995=CIRCLE('',#5302,7.24999999999999);
#1996=CIRCLE('',#5304,6.);
#1997=CIRCLE('',#5305,6.24999999999999);
#1998=CIRCLE('',#5307,6.);
#1999=CIRCLE('',#5308,6.);
#2000=CIRCLE('',#5310,6.24999999999999);
#2001=CIRCLE('',#5312,7.24999999999999);
#2002=CIRCLE('',#5314,7.24999999999999);
#2003=CIRCLE('',#5318,1.49484711634153);
#2004=CIRCLE('',#5320,10.5);
#2005=CIRCLE('',#5321,10.25);
#2006=CIRCLE('',#5323,9.25000000000001);
#2007=CIRCLE('',#5324,9.25);
#2008=CIRCLE('',#5326,1.49484711634153);
#2009=CIRCLE('',#5327,9.25);
#2010=CIRCLE('',#5329,9.25000000000001);
#2011=CIRCLE('',#5331,10.5);
#2012=CIRCLE('',#5332,10.5);
#2013=CIRCLE('',#5333,10.25);
#2014=CIRCLE('',#5338,1.49484711634153);
#2015=CIRCLE('',#5340,1.49484711634153);
#2016=CIRCLE('',#5342,1.49484711634153);
#2017=CIRCLE('',#5344,1.49484711634153);
#2018=CIRCLE('',#5346,1.49484711634153);
#2019=CIRCLE('',#5348,1.49484711634153);
#2020=CIRCLE('',#5350,1.49484711634153);
#2021=CIRCLE('',#5352,1.49484711634153);
#2022=CIRCLE('',#5354,1.49484711634153);
#2023=CIRCLE('',#5355,1.59062243825056);
#2024=CIRCLE('',#5356,1.42003545260829);
#2025=CIRCLE('',#5357,1.59062243825056);
#2026=CIRCLE('',#5359,1.49484711634152);
#2027=CIRCLE('',#5360,1.40874692590067);
#2028=CIRCLE('',#5361,1.40874692590067);
#2029=CIRCLE('',#5364,1.59062243825056);
#2030=CIRCLE('',#5365,1.42003545260833);
#2031=CIRCLE('',#5366,1.59062243825056);
#2032=CIRCLE('',#5368,1.49484711634152);
#2033=CIRCLE('',#5369,1.40874692590067);
#2034=CIRCLE('',#5370,1.40874692590067);
#2035=CIRCLE('',#5373,1.59062243825056);
#2036=CIRCLE('',#5374,1.42003545260828);
#2037=CIRCLE('',#5375,1.59062243825056);
#2038=CIRCLE('',#5377,1.49484711634152);
#2039=CIRCLE('',#5378,1.40874692590067);
#2040=CIRCLE('',#5379,1.40874692590067);
#2041=CIRCLE('',#5382,1.59062243825056);
#2042=CIRCLE('',#5383,1.4200354526083);
#2043=CIRCLE('',#5384,1.59062243825056);
#2044=CIRCLE('',#5386,1.49484711634152);
#2045=CIRCLE('',#5387,1.40874692590067);
#2046=CIRCLE('',#5388,1.40874692590067);
#2047=CIRCLE('',#5391,1.59062243825056);
#2048=CIRCLE('',#5392,1.42003545260827);
#2049=CIRCLE('',#5393,1.59062243825056);
#2050=CIRCLE('',#5395,1.49484711634152);
#2051=CIRCLE('',#5396,1.40874692590067);
#2052=CIRCLE('',#5397,1.40874692590067);
#2053=CIRCLE('',#5400,1.59062243825056);
#2054=CIRCLE('',#5401,1.42003545260833);
#2055=CIRCLE('',#5402,1.59062243825056);
#2056=CIRCLE('',#5404,1.49484711634152);
#2057=CIRCLE('',#5405,1.40874692590067);
#2058=CIRCLE('',#5406,1.40874692590067);
#2059=CIRCLE('',#5409,1.59062243825056);
#2060=CIRCLE('',#5410,1.42003545260831);
#2061=CIRCLE('',#5411,1.59062243825056);
#2062=CIRCLE('',#5413,1.49484711634152);
#2063=CIRCLE('',#5414,1.40874692590067);
#2064=CIRCLE('',#5415,1.40874692590067);
#2065=CIRCLE('',#5418,1.59062243825056);
#2066=CIRCLE('',#5419,1.42003545260829);
#2067=CIRCLE('',#5420,1.59062243825056);
#2068=CIRCLE('',#5422,1.49484711634152);
#2069=CIRCLE('',#5423,1.40874692590067);
#2070=CIRCLE('',#5424,1.40874692590067);
#2071=CIRCLE('',#5427,1.59062243825056);
#2072=CIRCLE('',#5428,1.42003545260828);
#2073=CIRCLE('',#5429,1.59062243825056);
#2074=CIRCLE('',#5431,1.49484711634152);
#2075=CIRCLE('',#5432,1.40874692590067);
#2076=CIRCLE('',#5433,1.40874692590067);
#2077=CIRCLE('',#5436,1.59062243825056);
#2078=CIRCLE('',#5437,1.42003545260832);
#2079=CIRCLE('',#5438,1.59062243825056);
#2080=CIRCLE('',#5440,1.49484711634152);
#2081=CIRCLE('',#5441,1.40874692590067);
#2082=CIRCLE('',#5442,1.40874692590067);
#2083=CIRCLE('',#5446,8.25);
#2084=CIRCLE('',#5447,8.25);
#2085=CIRCLE('',#5449,8.75);
#2086=CIRCLE('',#5450,8.75);
#2087=CIRCLE('',#5453,1.59062243825056);
#2088=CIRCLE('',#5454,1.42003545260827);
#2089=CIRCLE('',#5455,1.59062243825056);
#2090=CIRCLE('',#5457,1.49484711634152);
#2091=CIRCLE('',#5458,1.40874692590067);
#2092=CIRCLE('',#5459,1.40874692590067);
#2093=CIRCLE('',#5462,1.59062243825056);
#2094=CIRCLE('',#5463,1.42003545260827);
#2095=CIRCLE('',#5464,1.59062243825056);
#2096=CIRCLE('',#5466,1.49484711634152);
#2097=CIRCLE('',#5467,1.40874692590067);
#2098=CIRCLE('',#5468,1.40874692590067);
#2099=CIRCLE('',#5472,1.49484711634153);
#2100=CIRCLE('',#5474,1.49484711634153);
#2101=CIRCLE('',#5476,7.42777777777777);
#2102=CIRCLE('',#5477,0.0277777777777778);
#2103=CIRCLE('',#5478,7.39999999999999);
#2104=CIRCLE('',#5479,7.39999999999999);
#2105=CIRCLE('',#5481,9.1);
#2106=CIRCLE('',#5482,0.0277777777777778);
#2107=CIRCLE('',#5483,9.07222222222223);
#2108=CIRCLE('',#5484,9.1);
#2109=CIRCLE('',#5486,9.1);
#2110=CIRCLE('',#5487,9.1);
#2111=CIRCLE('',#5489,9.25000000000001);
#2112=CIRCLE('',#5491,7.24999999999999);
#2113=CIRCLE('',#5492,7.39999999999999);
#2114=CIRCLE('',#5497,9.1);
#2115=CIRCLE('',#5498,0.027777777777778);
#2116=CIRCLE('',#5499,9.07222222222222);
#2117=CIRCLE('',#5501,7.42777777777777);
#2118=CIRCLE('',#5502,0.027777777777778);
#2119=CIRCLE('',#5503,7.39999999999999);
#2120=CIRCLE('',#5505,7.39999999999999);
#2121=CIRCLE('',#5506,7.39999999999999);
#2122=CIRCLE('',#5508,7.24999999999999);
#2123=CIRCLE('',#5510,9.25);
#2124=CIRCLE('',#5511,9.1);
#2360=VERTEX_POINT('',#7825);
#2361=VERTEX_POINT('',#7827);
#2362=VERTEX_POINT('',#7831);
#2363=VERTEX_POINT('',#7833);
#2364=VERTEX_POINT('',#7837);
#2365=VERTEX_POINT('',#7839);
#2366=VERTEX_POINT('',#7843);
#2367=VERTEX_POINT('',#7847);
#2368=VERTEX_POINT('',#7851);
#2369=VERTEX_POINT('',#7857);
#2370=VERTEX_POINT('',#7858);
#2371=VERTEX_POINT('',#7861);
#2372=VERTEX_POINT('',#7863);
#2373=VERTEX_POINT('',#7867);
#2374=VERTEX_POINT('',#7869);
#2375=VERTEX_POINT('',#7873);
#2376=VERTEX_POINT('',#7877);
#2377=VERTEX_POINT('',#7881);
#2378=VERTEX_POINT('',#7882);
#2379=VERTEX_POINT('',#7885);
#2380=VERTEX_POINT('',#7893);
#2381=VERTEX_POINT('',#7894);
#2382=VERTEX_POINT('',#7897);
#2383=VERTEX_POINT('',#7898);
#2384=VERTEX_POINT('',#7901);
#2385=VERTEX_POINT('',#7902);
#2386=VERTEX_POINT('',#7905);
#2387=VERTEX_POINT('',#7906);
#2388=VERTEX_POINT('',#7909);
#2389=VERTEX_POINT('',#7910);
#2390=VERTEX_POINT('',#7913);
#2391=VERTEX_POINT('',#7914);
#2392=VERTEX_POINT('',#7917);
#2393=VERTEX_POINT('',#7918);
#2394=VERTEX_POINT('',#7921);
#2395=VERTEX_POINT('',#7922);
#2396=VERTEX_POINT('',#7925);
#2397=VERTEX_POINT('',#7926);
#2398=VERTEX_POINT('',#7955);
#2399=VERTEX_POINT('',#7957);
#2400=VERTEX_POINT('',#7961);
#2401=VERTEX_POINT('',#7962);
#2402=VERTEX_POINT('',#7964);
#2403=VERTEX_POINT('',#7966);
#2404=VERTEX_POINT('',#7997);
#2405=VERTEX_POINT('',#7999);
#2406=VERTEX_POINT('',#8003);
#2407=VERTEX_POINT('',#8004);
#2408=VERTEX_POINT('',#8006);
#2409=VERTEX_POINT('',#8008);
#2410=VERTEX_POINT('',#8039);
#2411=VERTEX_POINT('',#8041);
#2412=VERTEX_POINT('',#8045);
#2413=VERTEX_POINT('',#8046);
#2414=VERTEX_POINT('',#8048);
#2415=VERTEX_POINT('',#8050);
#2416=VERTEX_POINT('',#8081);
#2417=VERTEX_POINT('',#8083);
#2418=VERTEX_POINT('',#8087);
#2419=VERTEX_POINT('',#8088);
#2420=VERTEX_POINT('',#8090);
#2421=VERTEX_POINT('',#8092);
#2422=VERTEX_POINT('',#8123);
#2423=VERTEX_POINT('',#8125);
#2424=VERTEX_POINT('',#8129);
#2425=VERTEX_POINT('',#8130);
#2426=VERTEX_POINT('',#8132);
#2427=VERTEX_POINT('',#8134);
#2428=VERTEX_POINT('',#8165);
#2429=VERTEX_POINT('',#8167);
#2430=VERTEX_POINT('',#8171);
#2431=VERTEX_POINT('',#8172);
#2432=VERTEX_POINT('',#8174);
#2433=VERTEX_POINT('',#8176);
#2434=VERTEX_POINT('',#8207);
#2435=VERTEX_POINT('',#8209);
#2436=VERTEX_POINT('',#8213);
#2437=VERTEX_POINT('',#8214);
#2438=VERTEX_POINT('',#8216);
#2439=VERTEX_POINT('',#8218);
#2440=VERTEX_POINT('',#8249);
#2441=VERTEX_POINT('',#8251);
#2442=VERTEX_POINT('',#8255);
#2443=VERTEX_POINT('',#8256);
#2444=VERTEX_POINT('',#8258);
#2445=VERTEX_POINT('',#8260);
#2446=VERTEX_POINT('',#8291);
#2447=VERTEX_POINT('',#8293);
#2448=VERTEX_POINT('',#8297);
#2449=VERTEX_POINT('',#8298);
#2450=VERTEX_POINT('',#8300);
#2451=VERTEX_POINT('',#8302);
#2452=VERTEX_POINT('',#8333);
#2453=VERTEX_POINT('',#8335);
#2454=VERTEX_POINT('',#8339);
#2455=VERTEX_POINT('',#8340);
#2456=VERTEX_POINT('',#8342);
#2457=VERTEX_POINT('',#8344);
#2458=VERTEX_POINT('',#8349);
#2459=VERTEX_POINT('',#8351);
#2460=VERTEX_POINT('',#8355);
#2461=VERTEX_POINT('',#8357);
#2462=VERTEX_POINT('',#8389);
#2463=VERTEX_POINT('',#8391);
#2464=VERTEX_POINT('',#8395);
#2465=VERTEX_POINT('',#8396);
#2466=VERTEX_POINT('',#8398);
#2467=VERTEX_POINT('',#8400);
#2468=VERTEX_POINT('',#8431);
#2469=VERTEX_POINT('',#8433);
#2470=VERTEX_POINT('',#8437);
#2471=VERTEX_POINT('',#8438);
#2472=VERTEX_POINT('',#8440);
#2473=VERTEX_POINT('',#8442);
#2474=VERTEX_POINT('',#8447);
#2475=VERTEX_POINT('',#8448);
#2476=VERTEX_POINT('',#8451);
#2477=VERTEX_POINT('',#8452);
#2478=VERTEX_POINT('',#8455);
#2479=VERTEX_POINT('',#8457);
#2480=VERTEX_POINT('',#8459);
#2481=VERTEX_POINT('',#8463);
#2482=VERTEX_POINT('',#8464);
#2483=VERTEX_POINT('',#8466);
#2484=VERTEX_POINT('',#8471);
#2485=VERTEX_POINT('',#8472);
#2486=VERTEX_POINT('',#8477);
#2487=VERTEX_POINT('',#8481);
#2488=VERTEX_POINT('',#8483);
#2489=VERTEX_POINT('',#8491);
#2490=VERTEX_POINT('',#8493);
#2491=VERTEX_POINT('',#8497);
#2492=VERTEX_POINT('',#8499);
#2493=VERTEX_POINT('',#8503);
#2494=VERTEX_POINT('',#8504);
#2495=VERTEX_POINT('',#8509);
#2496=VERTEX_POINT('',#8513);
#2497=VERTEX_POINT('',#8515);
#2881=EDGE_CURVE('',#2360,#2360,#1993,.T.);
#2882=EDGE_CURVE('',#2360,#2361,#1994,.T.);
#2883=EDGE_CURVE('',#2361,#2361,#1995,.T.);
#2884=EDGE_CURVE('',#2362,#2362,#1996,.T.);
#2885=EDGE_CURVE('',#2362,#2363,#1515,.T.);
#2886=EDGE_CURVE('',#2363,#2363,#1997,.T.);
#2887=EDGE_CURVE('',#2362,#2364,#1516,.T.);
#2888=EDGE_CURVE('',#2364,#2365,#1998,.T.);
#2889=EDGE_CURVE('',#2365,#2364,#1999,.T.);
#2890=EDGE_CURVE('',#2365,#2366,#1517,.T.);
#2891=EDGE_CURVE('',#2366,#2366,#2000,.T.);
#2892=EDGE_CURVE('',#2367,#2367,#2001,.T.);
#2893=EDGE_CURVE('',#2367,#2361,#1518,.T.);
#2894=EDGE_CURVE('',#2360,#2368,#1519,.T.);
#2895=EDGE_CURVE('',#2368,#2368,#2002,.T.);
#2896=EDGE_CURVE('',#2369,#2370,#2003,.T.);
#2897=EDGE_CURVE('',#2371,#2371,#2004,.T.);
#2898=EDGE_CURVE('',#2371,#2372,#1520,.T.);
#2899=EDGE_CURVE('',#2372,#2372,#2005,.T.);
#2900=EDGE_CURVE('',#2373,#2373,#2006,.T.);
#2901=EDGE_CURVE('',#2373,#2374,#1521,.T.);
#2902=EDGE_CURVE('',#2374,#2374,#2007,.T.);
#2903=EDGE_CURVE('',#2373,#2375,#2008,.T.);
#2904=EDGE_CURVE('',#2375,#2375,#2009,.T.);
#2905=EDGE_CURVE('',#2376,#2376,#2010,.T.);
#2906=EDGE_CURVE('',#2376,#2375,#1522,.T.);
#2907=EDGE_CURVE('',#2377,#2378,#2011,.T.);
#2908=EDGE_CURVE('',#2378,#2377,#2012,.T.);
#2909=EDGE_CURVE('',#2378,#2379,#1523,.T.);
#2910=EDGE_CURVE('',#2379,#2379,#2013,.T.);
#2911=EDGE_CURVE('',#2371,#2377,#1524,.T.);
#2912=EDGE_CURVE('',#2380,#2381,#2014,.T.);
#2913=EDGE_CURVE('',#2382,#2383,#2015,.T.);
#2914=EDGE_CURVE('',#2384,#2385,#2016,.T.);
#2915=EDGE_CURVE('',#2386,#2387,#2017,.T.);
#2916=EDGE_CURVE('',#2388,#2389,#2018,.T.);
#2917=EDGE_CURVE('',#2390,#2391,#2019,.T.);
#2918=EDGE_CURVE('',#2392,#2393,#2020,.T.);
#2919=EDGE_CURVE('',#2394,#2395,#2021,.T.);
#2920=EDGE_CURVE('',#2396,#2397,#2022,.T.);
#2921=EDGE_CURVE('',#2398,#2398,#2023,.T.);
#2922=EDGE_CURVE('',#2398,#2399,#2024,.T.);
#2923=EDGE_CURVE('',#2399,#2399,#2025,.T.);
#2924=EDGE_CURVE('',#2400,#2401,#2026,.T.);
#2925=EDGE_CURVE('',#2402,#2402,#2027,.T.);
#2926=EDGE_CURVE('',#2403,#2403,#2028,.T.);
#2927=EDGE_CURVE('',#2404,#2404,#2029,.T.);
#2928=EDGE_CURVE('',#2404,#2405,#2030,.T.);
#2929=EDGE_CURVE('',#2405,#2405,#2031,.T.);
#2930=EDGE_CURVE('',#2406,#2407,#2032,.T.);
#2931=EDGE_CURVE('',#2408,#2408,#2033,.T.);
#2932=EDGE_CURVE('',#2409,#2409,#2034,.T.);
#2933=EDGE_CURVE('',#2410,#2410,#2035,.T.);
#2934=EDGE_CURVE('',#2410,#2411,#2036,.T.);
#2935=EDGE_CURVE('',#2411,#2411,#2037,.T.);
#2936=EDGE_CURVE('',#2412,#2413,#2038,.T.);
#2937=EDGE_CURVE('',#2414,#2414,#2039,.T.);
#2938=EDGE_CURVE('',#2415,#2415,#2040,.T.);
#2939=EDGE_CURVE('',#2416,#2416,#2041,.T.);
#2940=EDGE_CURVE('',#2416,#2417,#2042,.T.);
#2941=EDGE_CURVE('',#2417,#2417,#2043,.T.);
#2942=EDGE_CURVE('',#2418,#2419,#2044,.T.);
#2943=EDGE_CURVE('',#2420,#2420,#2045,.T.);
#2944=EDGE_CURVE('',#2421,#2421,#2046,.T.);
#2945=EDGE_CURVE('',#2422,#2422,#2047,.T.);
#2946=EDGE_CURVE('',#2422,#2423,#2048,.T.);
#2947=EDGE_CURVE('',#2423,#2423,#2049,.T.);
#2948=EDGE_CURVE('',#2424,#2425,#2050,.T.);
#2949=EDGE_CURVE('',#2426,#2426,#2051,.T.);
#2950=EDGE_CURVE('',#2427,#2427,#2052,.T.);
#2951=EDGE_CURVE('',#2428,#2428,#2053,.T.);
#2952=EDGE_CURVE('',#2428,#2429,#2054,.T.);
#2953=EDGE_CURVE('',#2429,#2429,#2055,.T.);
#2954=EDGE_CURVE('',#2430,#2431,#2056,.T.);
#2955=EDGE_CURVE('',#2432,#2432,#2057,.T.);
#2956=EDGE_CURVE('',#2433,#2433,#2058,.T.);
#2957=EDGE_CURVE('',#2434,#2434,#2059,.T.);
#2958=EDGE_CURVE('',#2434,#2435,#2060,.T.);
#2959=EDGE_CURVE('',#2435,#2435,#2061,.T.);
#2960=EDGE_CURVE('',#2436,#2437,#2062,.T.);
#2961=EDGE_CURVE('',#2438,#2438,#2063,.T.);
#2962=EDGE_CURVE('',#2439,#2439,#2064,.T.);
#2963=EDGE_CURVE('',#2440,#2440,#2065,.T.);
#2964=EDGE_CURVE('',#2440,#2441,#2066,.T.);
#2965=EDGE_CURVE('',#2441,#2441,#2067,.T.);
#2966=EDGE_CURVE('',#2442,#2443,#2068,.T.);
#2967=EDGE_CURVE('',#2444,#2444,#2069,.T.);
#2968=EDGE_CURVE('',#2445,#2445,#2070,.T.);
#2969=EDGE_CURVE('',#2446,#2446,#2071,.T.);
#2970=EDGE_CURVE('',#2446,#2447,#2072,.T.);
#2971=EDGE_CURVE('',#2447,#2447,#2073,.T.);
#2972=EDGE_CURVE('',#2448,#2449,#2074,.T.);
#2973=EDGE_CURVE('',#2450,#2450,#2075,.T.);
#2974=EDGE_CURVE('',#2451,#2451,#2076,.T.);
#2975=EDGE_CURVE('',#2452,#2452,#2077,.T.);
#2976=EDGE_CURVE('',#2452,#2453,#2078,.T.);
#2977=EDGE_CURVE('',#2453,#2453,#2079,.T.);
#2978=EDGE_CURVE('',#2454,#2455,#2080,.T.);
#2979=EDGE_CURVE('',#2456,#2456,#2081,.T.);
#2980=EDGE_CURVE('',#2457,#2457,#2082,.T.);
#2981=EDGE_CURVE('',#2458,#2458,#2083,.T.);
#2982=EDGE_CURVE('',#2458,#2459,#1525,.T.);
#2983=EDGE_CURVE('',#2459,#2459,#2084,.T.);
#2984=EDGE_CURVE('',#2460,#2460,#2085,.T.);
#2985=EDGE_CURVE('',#2460,#2461,#1526,.T.);
#2986=EDGE_CURVE('',#2461,#2461,#2086,.T.);
#2987=EDGE_CURVE('',#2462,#2462,#2087,.T.);
#2988=EDGE_CURVE('',#2462,#2463,#2088,.T.);
#2989=EDGE_CURVE('',#2463,#2463,#2089,.T.);
#2990=EDGE_CURVE('',#2464,#2465,#2090,.T.);
#2991=EDGE_CURVE('',#2466,#2466,#2091,.T.);
#2992=EDGE_CURVE('',#2467,#2467,#2092,.T.);
#2993=EDGE_CURVE('',#2468,#2468,#2093,.T.);
#2994=EDGE_CURVE('',#2468,#2469,#2094,.T.);
#2995=EDGE_CURVE('',#2469,#2469,#2095,.T.);
#2996=EDGE_CURVE('',#2470,#2471,#2096,.T.);
#2997=EDGE_CURVE('',#2472,#2472,#2097,.T.);
#2998=EDGE_CURVE('',#2473,#2473,#2098,.T.);
#2999=EDGE_CURVE('',#2474,#2475,#2099,.T.);
#3000=EDGE_CURVE('',#2476,#2477,#2100,.T.);
#3001=EDGE_CURVE('',#2478,#2478,#2101,.T.);
#3002=EDGE_CURVE('',#2478,#2479,#2102,.T.);
#3003=EDGE_CURVE('',#2479,#2480,#2103,.T.);
#3004=EDGE_CURVE('',#2480,#2479,#2104,.T.);
#3005=EDGE_CURVE('',#2481,#2482,#2105,.T.);
#3006=EDGE_CURVE('',#2482,#2483,#2106,.T.);
#3007=EDGE_CURVE('',#2483,#2483,#2107,.T.);
#3008=EDGE_CURVE('',#2482,#2481,#2108,.T.);
#3009=EDGE_CURVE('',#2484,#2485,#2109,.T.);
#3010=EDGE_CURVE('',#2485,#2484,#2110,.T.);
#3011=EDGE_CURVE('',#2485,#2481,#1527,.T.);
#3012=EDGE_CURVE('',#2486,#2486,#2111,.T.);
#3013=EDGE_CURVE('',#2486,#2484,#1528,.T.);
#3014=EDGE_CURVE('',#2487,#2487,#2112,.T.);
#3015=EDGE_CURVE('',#2487,#2488,#1529,.T.);
#3016=EDGE_CURVE('',#2488,#2488,#2113,.T.);
#3017=EDGE_CURVE('',#2480,#2488,#1530,.T.);
#3018=EDGE_CURVE('',#2489,#2489,#2114,.T.);
#3019=EDGE_CURVE('',#2489,#2490,#2115,.T.);
#3020=EDGE_CURVE('',#2490,#2490,#2116,.T.);
#3021=EDGE_CURVE('',#2491,#2491,#2117,.T.);
#3022=EDGE_CURVE('',#2491,#2492,#2118,.T.);
#3023=EDGE_CURVE('',#2492,#2492,#2119,.T.);
#3024=EDGE_CURVE('',#2493,#2494,#2120,.T.);
#3025=EDGE_CURVE('',#2494,#2493,#2121,.T.);
#3026=EDGE_CURVE('',#2494,#2492,#1531,.T.);
#3027=EDGE_CURVE('',#2495,#2495,#2122,.T.);
#3028=EDGE_CURVE('',#2495,#2493,#1532,.T.);
#3029=EDGE_CURVE('',#2496,#2496,#2123,.T.);
#3030=EDGE_CURVE('',#2496,#2497,#1533,.T.);
#3031=EDGE_CURVE('',#2497,#2497,#2124,.T.);
#3032=EDGE_CURVE('',#2489,#2497,#1534,.T.);
#3657=ORIENTED_EDGE('',*,*,#2881,.T.);
#3658=ORIENTED_EDGE('',*,*,#2882,.T.);
#3659=ORIENTED_EDGE('',*,*,#2883,.F.);
#3660=ORIENTED_EDGE('',*,*,#2882,.F.);
#3661=ORIENTED_EDGE('',*,*,#2884,.T.);
#3662=ORIENTED_EDGE('',*,*,#2885,.T.);
#3663=ORIENTED_EDGE('',*,*,#2886,.F.);
#3664=ORIENTED_EDGE('',*,*,#2885,.F.);
#3665=ORIENTED_EDGE('',*,*,#2884,.F.);
#3666=ORIENTED_EDGE('',*,*,#2887,.T.);
#3667=ORIENTED_EDGE('',*,*,#2888,.T.);
#3668=ORIENTED_EDGE('',*,*,#2889,.T.);
#3669=ORIENTED_EDGE('',*,*,#2887,.F.);
#3670=ORIENTED_EDGE('',*,*,#2889,.F.);
#3671=ORIENTED_EDGE('',*,*,#2890,.T.);
#3672=ORIENTED_EDGE('',*,*,#2891,.T.);
#3673=ORIENTED_EDGE('',*,*,#2890,.F.);
#3674=ORIENTED_EDGE('',*,*,#2888,.F.);
#3675=ORIENTED_EDGE('',*,*,#2892,.F.);
#3676=ORIENTED_EDGE('',*,*,#2893,.T.);
#3677=ORIENTED_EDGE('',*,*,#2883,.T.);
#3678=ORIENTED_EDGE('',*,*,#2893,.F.);
#3679=ORIENTED_EDGE('',*,*,#2881,.F.);
#3680=ORIENTED_EDGE('',*,*,#2894,.T.);
#3681=ORIENTED_EDGE('',*,*,#2895,.T.);
#3682=ORIENTED_EDGE('',*,*,#2894,.F.);
#3683=ORIENTED_EDGE('',*,*,#2895,.F.);
#3684=ORIENTED_EDGE('',*,*,#2886,.T.);
#3685=ORIENTED_EDGE('',*,*,#2892,.T.);
#3686=ORIENTED_EDGE('',*,*,#2891,.F.);
#3687=ORIENTED_EDGE('',*,*,#2896,.T.);
#3688=ORIENTED_EDGE('',*,*,#2896,.F.);
#3689=ORIENTED_EDGE('',*,*,#2897,.T.);
#3690=ORIENTED_EDGE('',*,*,#2898,.T.);
#3691=ORIENTED_EDGE('',*,*,#2899,.F.);
#3692=ORIENTED_EDGE('',*,*,#2898,.F.);
#3693=ORIENTED_EDGE('',*,*,#2900,.F.);
#3694=ORIENTED_EDGE('',*,*,#2901,.T.);
#3695=ORIENTED_EDGE('',*,*,#2902,.T.);
#3696=ORIENTED_EDGE('',*,*,#2901,.F.);
#3697=ORIENTED_EDGE('',*,*,#2900,.T.);
#3698=ORIENTED_EDGE('',*,*,#2903,.T.);
#3699=ORIENTED_EDGE('',*,*,#2904,.F.);
#3700=ORIENTED_EDGE('',*,*,#2903,.F.);
#3701=ORIENTED_EDGE('',*,*,#2905,.F.);
#3702=ORIENTED_EDGE('',*,*,#2906,.T.);
#3703=ORIENTED_EDGE('',*,*,#2904,.T.);
#3704=ORIENTED_EDGE('',*,*,#2906,.F.);
#3705=ORIENTED_EDGE('',*,*,#2907,.F.);
#3706=ORIENTED_EDGE('',*,*,#2908,.F.);
#3707=ORIENTED_EDGE('',*,*,#2909,.T.);
#3708=ORIENTED_EDGE('',*,*,#2910,.T.);
#3709=ORIENTED_EDGE('',*,*,#2909,.F.);
#3710=ORIENTED_EDGE('',*,*,#2897,.F.);
#3711=ORIENTED_EDGE('',*,*,#2911,.T.);
#3712=ORIENTED_EDGE('',*,*,#2907,.T.);
#3713=ORIENTED_EDGE('',*,*,#2908,.T.);
#3714=ORIENTED_EDGE('',*,*,#2911,.F.);
#3715=ORIENTED_EDGE('',*,*,#2910,.F.);
#3716=ORIENTED_EDGE('',*,*,#2905,.T.);
#3717=ORIENTED_EDGE('',*,*,#2899,.T.);
#3718=ORIENTED_EDGE('',*,*,#2902,.F.);
#3719=ORIENTED_EDGE('',*,*,#2912,.T.);
#3720=ORIENTED_EDGE('',*,*,#2912,.F.);
#3721=ORIENTED_EDGE('',*,*,#2913,.T.);
#3722=ORIENTED_EDGE('',*,*,#2913,.F.);
#3723=ORIENTED_EDGE('',*,*,#2914,.T.);
#3724=ORIENTED_EDGE('',*,*,#2914,.F.);
#3725=ORIENTED_EDGE('',*,*,#2915,.T.);
#3726=ORIENTED_EDGE('',*,*,#2915,.F.);
#3727=ORIENTED_EDGE('',*,*,#2916,.T.);
#3728=ORIENTED_EDGE('',*,*,#2916,.F.);
#3729=ORIENTED_EDGE('',*,*,#2917,.T.);
#3730=ORIENTED_EDGE('',*,*,#2917,.F.);
#3731=ORIENTED_EDGE('',*,*,#2918,.T.);
#3732=ORIENTED_EDGE('',*,*,#2918,.F.);
#3733=ORIENTED_EDGE('',*,*,#2919,.T.);
#3734=ORIENTED_EDGE('',*,*,#2919,.F.);
#3735=ORIENTED_EDGE('',*,*,#2920,.T.);
#3736=ORIENTED_EDGE('',*,*,#2920,.F.);
#3737=ORIENTED_EDGE('',*,*,#2921,.F.);
#3738=ORIENTED_EDGE('',*,*,#2922,.T.);
#3739=ORIENTED_EDGE('',*,*,#2923,.T.);
#3740=ORIENTED_EDGE('',*,*,#2922,.F.);
#3741=ORIENTED_EDGE('',*,*,#2924,.T.);
#3742=ORIENTED_EDGE('',*,*,#2924,.F.);
#3743=ORIENTED_EDGE('',*,*,#2925,.T.);
#3744=ORIENTED_EDGE('',*,*,#2926,.F.);
#3745=ORIENTED_EDGE('',*,*,#2923,.F.);
#3746=ORIENTED_EDGE('',*,*,#2926,.T.);
#3747=ORIENTED_EDGE('',*,*,#2921,.T.);
#3748=ORIENTED_EDGE('',*,*,#2925,.F.);
#3749=ORIENTED_EDGE('',*,*,#2927,.F.);
#3750=ORIENTED_EDGE('',*,*,#2928,.T.);
#3751=ORIENTED_EDGE('',*,*,#2929,.T.);
#3752=ORIENTED_EDGE('',*,*,#2928,.F.);
#3753=ORIENTED_EDGE('',*,*,#2930,.T.);
#3754=ORIENTED_EDGE('',*,*,#2930,.F.);
#3755=ORIENTED_EDGE('',*,*,#2931,.T.);
#3756=ORIENTED_EDGE('',*,*,#2932,.F.);
#3757=ORIENTED_EDGE('',*,*,#2929,.F.);
#3758=ORIENTED_EDGE('',*,*,#2932,.T.);
#3759=ORIENTED_EDGE('',*,*,#2927,.T.);
#3760=ORIENTED_EDGE('',*,*,#2931,.F.);
#3761=ORIENTED_EDGE('',*,*,#2933,.F.);
#3762=ORIENTED_EDGE('',*,*,#2934,.T.);
#3763=ORIENTED_EDGE('',*,*,#2935,.T.);
#3764=ORIENTED_EDGE('',*,*,#2934,.F.);
#3765=ORIENTED_EDGE('',*,*,#2936,.T.);
#3766=ORIENTED_EDGE('',*,*,#2936,.F.);
#3767=ORIENTED_EDGE('',*,*,#2937,.T.);
#3768=ORIENTED_EDGE('',*,*,#2938,.F.);
#3769=ORIENTED_EDGE('',*,*,#2935,.F.);
#3770=ORIENTED_EDGE('',*,*,#2938,.T.);
#3771=ORIENTED_EDGE('',*,*,#2933,.T.);
#3772=ORIENTED_EDGE('',*,*,#2937,.F.);
#3773=ORIENTED_EDGE('',*,*,#2939,.F.);
#3774=ORIENTED_EDGE('',*,*,#2940,.T.);
#3775=ORIENTED_EDGE('',*,*,#2941,.T.);
#3776=ORIENTED_EDGE('',*,*,#2940,.F.);
#3777=ORIENTED_EDGE('',*,*,#2942,.T.);
#3778=ORIENTED_EDGE('',*,*,#2942,.F.);
#3779=ORIENTED_EDGE('',*,*,#2943,.T.);
#3780=ORIENTED_EDGE('',*,*,#2944,.F.);
#3781=ORIENTED_EDGE('',*,*,#2941,.F.);
#3782=ORIENTED_EDGE('',*,*,#2944,.T.);
#3783=ORIENTED_EDGE('',*,*,#2939,.T.);
#3784=ORIENTED_EDGE('',*,*,#2943,.F.);
#3785=ORIENTED_EDGE('',*,*,#2945,.F.);
#3786=ORIENTED_EDGE('',*,*,#2946,.T.);
#3787=ORIENTED_EDGE('',*,*,#2947,.T.);
#3788=ORIENTED_EDGE('',*,*,#2946,.F.);
#3789=ORIENTED_EDGE('',*,*,#2948,.T.);
#3790=ORIENTED_EDGE('',*,*,#2948,.F.);
#3791=ORIENTED_EDGE('',*,*,#2949,.T.);
#3792=ORIENTED_EDGE('',*,*,#2950,.F.);
#3793=ORIENTED_EDGE('',*,*,#2947,.F.);
#3794=ORIENTED_EDGE('',*,*,#2950,.T.);
#3795=ORIENTED_EDGE('',*,*,#2945,.T.);
#3796=ORIENTED_EDGE('',*,*,#2949,.F.);
#3797=ORIENTED_EDGE('',*,*,#2951,.F.);
#3798=ORIENTED_EDGE('',*,*,#2952,.T.);
#3799=ORIENTED_EDGE('',*,*,#2953,.T.);
#3800=ORIENTED_EDGE('',*,*,#2952,.F.);
#3801=ORIENTED_EDGE('',*,*,#2954,.T.);
#3802=ORIENTED_EDGE('',*,*,#2954,.F.);
#3803=ORIENTED_EDGE('',*,*,#2955,.T.);
#3804=ORIENTED_EDGE('',*,*,#2956,.F.);
#3805=ORIENTED_EDGE('',*,*,#2953,.F.);
#3806=ORIENTED_EDGE('',*,*,#2956,.T.);
#3807=ORIENTED_EDGE('',*,*,#2951,.T.);
#3808=ORIENTED_EDGE('',*,*,#2955,.F.);
#3809=ORIENTED_EDGE('',*,*,#2957,.F.);
#3810=ORIENTED_EDGE('',*,*,#2958,.T.);
#3811=ORIENTED_EDGE('',*,*,#2959,.T.);
#3812=ORIENTED_EDGE('',*,*,#2958,.F.);
#3813=ORIENTED_EDGE('',*,*,#2960,.T.);
#3814=ORIENTED_EDGE('',*,*,#2960,.F.);
#3815=ORIENTED_EDGE('',*,*,#2961,.T.);
#3816=ORIENTED_EDGE('',*,*,#2962,.F.);
#3817=ORIENTED_EDGE('',*,*,#2959,.F.);
#3818=ORIENTED_EDGE('',*,*,#2962,.T.);
#3819=ORIENTED_EDGE('',*,*,#2957,.T.);
#3820=ORIENTED_EDGE('',*,*,#2961,.F.);
#3821=ORIENTED_EDGE('',*,*,#2963,.F.);
#3822=ORIENTED_EDGE('',*,*,#2964,.T.);
#3823=ORIENTED_EDGE('',*,*,#2965,.T.);
#3824=ORIENTED_EDGE('',*,*,#2964,.F.);
#3825=ORIENTED_EDGE('',*,*,#2966,.T.);
#3826=ORIENTED_EDGE('',*,*,#2966,.F.);
#3827=ORIENTED_EDGE('',*,*,#2967,.T.);
#3828=ORIENTED_EDGE('',*,*,#2968,.F.);
#3829=ORIENTED_EDGE('',*,*,#2965,.F.);
#3830=ORIENTED_EDGE('',*,*,#2968,.T.);
#3831=ORIENTED_EDGE('',*,*,#2963,.T.);
#3832=ORIENTED_EDGE('',*,*,#2967,.F.);
#3833=ORIENTED_EDGE('',*,*,#2969,.F.);
#3834=ORIENTED_EDGE('',*,*,#2970,.T.);
#3835=ORIENTED_EDGE('',*,*,#2971,.T.);
#3836=ORIENTED_EDGE('',*,*,#2970,.F.);
#3837=ORIENTED_EDGE('',*,*,#2972,.T.);
#3838=ORIENTED_EDGE('',*,*,#2972,.F.);
#3839=ORIENTED_EDGE('',*,*,#2973,.T.);
#3840=ORIENTED_EDGE('',*,*,#2974,.F.);
#3841=ORIENTED_EDGE('',*,*,#2971,.F.);
#3842=ORIENTED_EDGE('',*,*,#2974,.T.);
#3843=ORIENTED_EDGE('',*,*,#2969,.T.);
#3844=ORIENTED_EDGE('',*,*,#2973,.F.);
#3845=ORIENTED_EDGE('',*,*,#2975,.F.);
#3846=ORIENTED_EDGE('',*,*,#2976,.T.);
#3847=ORIENTED_EDGE('',*,*,#2977,.T.);
#3848=ORIENTED_EDGE('',*,*,#2976,.F.);
#3849=ORIENTED_EDGE('',*,*,#2978,.T.);
#3850=ORIENTED_EDGE('',*,*,#2978,.F.);
#3851=ORIENTED_EDGE('',*,*,#2979,.T.);
#3852=ORIENTED_EDGE('',*,*,#2980,.F.);
#3853=ORIENTED_EDGE('',*,*,#2977,.F.);
#3854=ORIENTED_EDGE('',*,*,#2980,.T.);
#3855=ORIENTED_EDGE('',*,*,#2975,.T.);
#3856=ORIENTED_EDGE('',*,*,#2979,.F.);
#3857=ORIENTED_EDGE('',*,*,#2981,.T.);
#3858=ORIENTED_EDGE('',*,*,#2982,.T.);
#3859=ORIENTED_EDGE('',*,*,#2983,.F.);
#3860=ORIENTED_EDGE('',*,*,#2982,.F.);
#3861=ORIENTED_EDGE('',*,*,#2984,.T.);
#3862=ORIENTED_EDGE('',*,*,#2985,.T.);
#3863=ORIENTED_EDGE('',*,*,#2986,.F.);
#3864=ORIENTED_EDGE('',*,*,#2985,.F.);
#3865=ORIENTED_EDGE('',*,*,#2984,.F.);
#3866=ORIENTED_EDGE('',*,*,#2983,.T.);
#3867=ORIENTED_EDGE('',*,*,#2986,.T.);
#3868=ORIENTED_EDGE('',*,*,#2981,.F.);
#3869=ORIENTED_EDGE('',*,*,#2987,.F.);
#3870=ORIENTED_EDGE('',*,*,#2988,.T.);
#3871=ORIENTED_EDGE('',*,*,#2989,.T.);
#3872=ORIENTED_EDGE('',*,*,#2988,.F.);
#3873=ORIENTED_EDGE('',*,*,#2990,.T.);
#3874=ORIENTED_EDGE('',*,*,#2990,.F.);
#3875=ORIENTED_EDGE('',*,*,#2991,.T.);
#3876=ORIENTED_EDGE('',*,*,#2992,.F.);
#3877=ORIENTED_EDGE('',*,*,#2989,.F.);
#3878=ORIENTED_EDGE('',*,*,#2992,.T.);
#3879=ORIENTED_EDGE('',*,*,#2987,.T.);
#3880=ORIENTED_EDGE('',*,*,#2991,.F.);
#3881=ORIENTED_EDGE('',*,*,#2993,.F.);
#3882=ORIENTED_EDGE('',*,*,#2994,.T.);
#3883=ORIENTED_EDGE('',*,*,#2995,.T.);
#3884=ORIENTED_EDGE('',*,*,#2994,.F.);
#3885=ORIENTED_EDGE('',*,*,#2996,.T.);
#3886=ORIENTED_EDGE('',*,*,#2996,.F.);
#3887=ORIENTED_EDGE('',*,*,#2997,.T.);
#3888=ORIENTED_EDGE('',*,*,#2998,.F.);
#3889=ORIENTED_EDGE('',*,*,#2995,.F.);
#3890=ORIENTED_EDGE('',*,*,#2998,.T.);
#3891=ORIENTED_EDGE('',*,*,#2993,.T.);
#3892=ORIENTED_EDGE('',*,*,#2997,.F.);
#3893=ORIENTED_EDGE('',*,*,#2999,.T.);
#3894=ORIENTED_EDGE('',*,*,#2999,.F.);
#3895=ORIENTED_EDGE('',*,*,#3000,.T.);
#3896=ORIENTED_EDGE('',*,*,#3000,.F.);
#3897=ORIENTED_EDGE('',*,*,#3001,.T.);
#3898=ORIENTED_EDGE('',*,*,#3002,.T.);
#3899=ORIENTED_EDGE('',*,*,#3003,.T.);
#3900=ORIENTED_EDGE('',*,*,#3004,.T.);
#3901=ORIENTED_EDGE('',*,*,#3002,.F.);
#3902=ORIENTED_EDGE('',*,*,#3005,.T.);
#3903=ORIENTED_EDGE('',*,*,#3006,.T.);
#3904=ORIENTED_EDGE('',*,*,#3007,.T.);
#3905=ORIENTED_EDGE('',*,*,#3006,.F.);
#3906=ORIENTED_EDGE('',*,*,#3008,.T.);
#3907=ORIENTED_EDGE('',*,*,#3009,.F.);
#3908=ORIENTED_EDGE('',*,*,#3010,.F.);
#3909=ORIENTED_EDGE('',*,*,#3011,.T.);
#3910=ORIENTED_EDGE('',*,*,#3008,.F.);
#3911=ORIENTED_EDGE('',*,*,#3005,.F.);
#3912=ORIENTED_EDGE('',*,*,#3011,.F.);
#3913=ORIENTED_EDGE('',*,*,#3012,.F.);
#3914=ORIENTED_EDGE('',*,*,#3013,.T.);
#3915=ORIENTED_EDGE('',*,*,#3009,.T.);
#3916=ORIENTED_EDGE('',*,*,#3010,.T.);
#3917=ORIENTED_EDGE('',*,*,#3013,.F.);
#3918=ORIENTED_EDGE('',*,*,#3014,.T.);
#3919=ORIENTED_EDGE('',*,*,#3015,.T.);
#3920=ORIENTED_EDGE('',*,*,#3016,.F.);
#3921=ORIENTED_EDGE('',*,*,#3015,.F.);
#3922=ORIENTED_EDGE('',*,*,#3004,.F.);
#3923=ORIENTED_EDGE('',*,*,#3017,.T.);
#3924=ORIENTED_EDGE('',*,*,#3016,.T.);
#3925=ORIENTED_EDGE('',*,*,#3017,.F.);
#3926=ORIENTED_EDGE('',*,*,#3003,.F.);
#3927=ORIENTED_EDGE('',*,*,#3007,.F.);
#3928=ORIENTED_EDGE('',*,*,#3001,.F.);
#3929=ORIENTED_EDGE('',*,*,#3012,.T.);
#3930=ORIENTED_EDGE('',*,*,#3014,.F.);
#3931=ORIENTED_EDGE('',*,*,#3018,.T.);
#3932=ORIENTED_EDGE('',*,*,#3019,.T.);
#3933=ORIENTED_EDGE('',*,*,#3020,.T.);
#3934=ORIENTED_EDGE('',*,*,#3019,.F.);
#3935=ORIENTED_EDGE('',*,*,#3021,.T.);
#3936=ORIENTED_EDGE('',*,*,#3022,.T.);
#3937=ORIENTED_EDGE('',*,*,#3023,.T.);
#3938=ORIENTED_EDGE('',*,*,#3022,.F.);
#3939=ORIENTED_EDGE('',*,*,#3024,.F.);
#3940=ORIENTED_EDGE('',*,*,#3025,.F.);
#3941=ORIENTED_EDGE('',*,*,#3026,.T.);
#3942=ORIENTED_EDGE('',*,*,#3023,.F.);
#3943=ORIENTED_EDGE('',*,*,#3026,.F.);
#3944=ORIENTED_EDGE('',*,*,#3027,.F.);
#3945=ORIENTED_EDGE('',*,*,#3028,.T.);
#3946=ORIENTED_EDGE('',*,*,#3024,.T.);
#3947=ORIENTED_EDGE('',*,*,#3025,.T.);
#3948=ORIENTED_EDGE('',*,*,#3028,.F.);
#3949=ORIENTED_EDGE('',*,*,#3029,.T.);
#3950=ORIENTED_EDGE('',*,*,#3030,.T.);
#3951=ORIENTED_EDGE('',*,*,#3031,.F.);
#3952=ORIENTED_EDGE('',*,*,#3030,.F.);
#3953=ORIENTED_EDGE('',*,*,#3018,.F.);
#3954=ORIENTED_EDGE('',*,*,#3032,.T.);
#3955=ORIENTED_EDGE('',*,*,#3031,.T.);
#3956=ORIENTED_EDGE('',*,*,#3032,.F.);
#3957=ORIENTED_EDGE('',*,*,#3029,.F.);
#3958=ORIENTED_EDGE('',*,*,#3027,.T.);
#3959=ORIENTED_EDGE('',*,*,#3020,.F.);
#3960=ORIENTED_EDGE('',*,*,#3021,.F.);
#4589=CYLINDRICAL_SURFACE('',#5306,6.);
#4590=CYLINDRICAL_SURFACE('',#5311,7.24999999999999);
#4591=CYLINDRICAL_SURFACE('',#5313,7.24999999999999);
#4592=CYLINDRICAL_SURFACE('',#5322,9.25000000000001);
#4593=CYLINDRICAL_SURFACE('',#5328,9.25);
#4594=CYLINDRICAL_SURFACE('',#5334,10.5);
#4595=CYLINDRICAL_SURFACE('',#5445,8.25);
#4596=CYLINDRICAL_SURFACE('',#5448,8.75);
#4597=CYLINDRICAL_SURFACE('',#5485,9.1);
#4598=CYLINDRICAL_SURFACE('',#5493,7.39999999999999);
#4599=CYLINDRICAL_SURFACE('',#5504,7.39999999999999);
#4600=CYLINDRICAL_SURFACE('',#5512,9.1);
#4720=ADVANCED_FACE('',(#709),#124,.F.);
#4721=ADVANCED_FACE('',(#710),#107,.F.);
#4722=ADVANCED_FACE('',(#711),#4589,.F.);
#4723=ADVANCED_FACE('',(#712),#108,.F.);
#4724=ADVANCED_FACE('',(#713),#4590,.T.);
#4725=ADVANCED_FACE('',(#714),#4591,.T.);
#4726=ADVANCED_FACE('',(#715,#354),#511,.T.);
#4727=ADVANCED_FACE('',(#716,#355),#512,.T.);
#4728=ADVANCED_FACE('',(#717),#293,.T.);
#4729=ADVANCED_FACE('',(#718),#109,.T.);
#4730=ADVANCED_FACE('',(#719),#4592,.F.);
#4731=ADVANCED_FACE('',(#720),#125,.F.);
#4732=ADVANCED_FACE('',(#721),#4593,.F.);
#4733=ADVANCED_FACE('',(#722),#110,.T.);
#4734=ADVANCED_FACE('',(#723),#4594,.T.);
#4735=ADVANCED_FACE('',(#724,#356),#513,.T.);
#4736=ADVANCED_FACE('',(#725,#357),#514,.T.);
#4737=ADVANCED_FACE('',(#726),#294,.T.);
#4738=ADVANCED_FACE('',(#727),#295,.T.);
#4739=ADVANCED_FACE('',(#728),#296,.T.);
#4740=ADVANCED_FACE('',(#729),#297,.T.);
#4741=ADVANCED_FACE('',(#730),#298,.T.);
#4742=ADVANCED_FACE('',(#731),#299,.T.);
#4743=ADVANCED_FACE('',(#732),#300,.T.);
#4744=ADVANCED_FACE('',(#733),#301,.T.);
#4745=ADVANCED_FACE('',(#734),#302,.T.);
#4746=ADVANCED_FACE('',(#735),#95,.F.);
#4747=ADVANCED_FACE('',(#736,#358,#359),#303,.F.);
#4748=ADVANCED_FACE('',(#737,#360),#515,.F.);
#4749=ADVANCED_FACE('',(#738,#361),#516,.F.);
#4750=ADVANCED_FACE('',(#739),#96,.F.);
#4751=ADVANCED_FACE('',(#740,#362,#363),#304,.F.);
#4752=ADVANCED_FACE('',(#741,#364),#517,.F.);
#4753=ADVANCED_FACE('',(#742,#365),#518,.F.);
#4754=ADVANCED_FACE('',(#743),#97,.F.);
#4755=ADVANCED_FACE('',(#744,#366,#367),#305,.F.);
#4756=ADVANCED_FACE('',(#745,#368),#519,.F.);
#4757=ADVANCED_FACE('',(#746,#369),#520,.F.);
#4758=ADVANCED_FACE('',(#747),#98,.F.);
#4759=ADVANCED_FACE('',(#748,#370,#371),#306,.F.);
#4760=ADVANCED_FACE('',(#749,#372),#521,.F.);
#4761=ADVANCED_FACE('',(#750,#373),#522,.F.);
#4762=ADVANCED_FACE('',(#751),#99,.F.);
#4763=ADVANCED_FACE('',(#752,#374,#375),#307,.F.);
#4764=ADVANCED_FACE('',(#753,#376),#523,.F.);
#4765=ADVANCED_FACE('',(#754,#377),#524,.F.);
#4766=ADVANCED_FACE('',(#755),#100,.F.);
#4767=ADVANCED_FACE('',(#756,#378,#379),#308,.F.);
#4768=ADVANCED_FACE('',(#757,#380),#525,.F.);
#4769=ADVANCED_FACE('',(#758,#381),#526,.F.);
#4770=ADVANCED_FACE('',(#759),#101,.F.);
#4771=ADVANCED_FACE('',(#760,#382,#383),#309,.F.);
#4772=ADVANCED_FACE('',(#761,#384),#527,.F.);
#4773=ADVANCED_FACE('',(#762,#385),#528,.F.);
#4774=ADVANCED_FACE('',(#763),#102,.F.);
#4775=ADVANCED_FACE('',(#764,#386,#387),#310,.F.);
#4776=ADVANCED_FACE('',(#765,#388),#529,.F.);
#4777=ADVANCED_FACE('',(#766,#389),#530,.F.);
#4778=ADVANCED_FACE('',(#767),#103,.F.);
#4779=ADVANCED_FACE('',(#768,#390,#391),#311,.F.);
#4780=ADVANCED_FACE('',(#769,#392),#531,.F.);
#4781=ADVANCED_FACE('',(#770,#393),#532,.F.);
#4782=ADVANCED_FACE('',(#771),#104,.F.);
#4783=ADVANCED_FACE('',(#772,#394,#395),#312,.F.);
#4784=ADVANCED_FACE('',(#773,#396),#533,.F.);
#4785=ADVANCED_FACE('',(#774,#397),#534,.F.);
#4786=ADVANCED_FACE('',(#775),#4595,.F.);
#4787=ADVANCED_FACE('',(#776),#4596,.T.);
#4788=ADVANCED_FACE('',(#777,#398),#535,.F.);
#4789=ADVANCED_FACE('',(#778,#399),#536,.T.);
#4790=ADVANCED_FACE('',(#779),#105,.F.);
#4791=ADVANCED_FACE('',(#780,#400,#401),#313,.F.);
#4792=ADVANCED_FACE('',(#781,#402),#537,.F.);
#4793=ADVANCED_FACE('',(#782,#403),#538,.F.);
#4794=ADVANCED_FACE('',(#783),#106,.F.);
#4795=ADVANCED_FACE('',(#784,#404,#405),#314,.F.);
#4796=ADVANCED_FACE('',(#785,#406),#539,.F.);
#4797=ADVANCED_FACE('',(#786,#407),#540,.F.);
#4798=ADVANCED_FACE('',(#787),#315,.T.);
#4799=ADVANCED_FACE('',(#788),#316,.T.);
#4800=ADVANCED_FACE('',(#789),#126,.T.);
#4801=ADVANCED_FACE('',(#790),#127,.T.);
#4802=ADVANCED_FACE('',(#791),#4597,.T.);
#4803=ADVANCED_FACE('',(#792),#111,.T.);
#4804=ADVANCED_FACE('',(#793),#112,.F.);
#4805=ADVANCED_FACE('',(#794),#4598,.F.);
#4806=ADVANCED_FACE('',(#795,#408),#541,.T.);
#4807=ADVANCED_FACE('',(#796,#409),#542,.T.);
#4808=ADVANCED_FACE('',(#797),#128,.T.);
#4809=ADVANCED_FACE('',(#798),#129,.T.);
#4810=ADVANCED_FACE('',(#799),#4599,.F.);
#4811=ADVANCED_FACE('',(#800),#113,.F.);
#4812=ADVANCED_FACE('',(#801),#114,.T.);
#4813=ADVANCED_FACE('',(#802),#4600,.T.);
#4814=ADVANCED_FACE('',(#803,#410),#543,.T.);
#4815=ADVANCED_FACE('',(#804,#411),#544,.T.);
#4967=CLOSED_SHELL('',(#4720,#4721,#4722,#4723,#4724,#4725,#4726,#4727));
#4968=CLOSED_SHELL('',(#4728));
#4969=CLOSED_SHELL('',(#4729,#4730,#4731,#4732,#4733,#4734,#4735,#4736));
#4970=CLOSED_SHELL('',(#4737));
#4971=CLOSED_SHELL('',(#4738));
#4972=CLOSED_SHELL('',(#4739));
#4973=CLOSED_SHELL('',(#4740));
#4974=CLOSED_SHELL('',(#4741));
#4975=CLOSED_SHELL('',(#4742));
#4976=CLOSED_SHELL('',(#4743));
#4977=CLOSED_SHELL('',(#4744));
#4978=CLOSED_SHELL('',(#4745));
#4979=CLOSED_SHELL('',(#4746,#4747,#4748,#4749));
#4980=CLOSED_SHELL('',(#4750,#4751,#4752,#4753));
#4981=CLOSED_SHELL('',(#4754,#4755,#4756,#4757));
#4982=CLOSED_SHELL('',(#4758,#4759,#4760,#4761));
#4983=CLOSED_SHELL('',(#4762,#4763,#4764,#4765));
#4984=CLOSED_SHELL('',(#4766,#4767,#4768,#4769));
#4985=CLOSED_SHELL('',(#4770,#4771,#4772,#4773));
#4986=CLOSED_SHELL('',(#4774,#4775,#4776,#4777));
#4987=CLOSED_SHELL('',(#4778,#4779,#4780,#4781));
#4988=CLOSED_SHELL('',(#4782,#4783,#4784,#4785));
#4989=CLOSED_SHELL('',(#4786,#4787,#4788,#4789));
#4990=CLOSED_SHELL('',(#4790,#4791,#4792,#4793));
#4991=CLOSED_SHELL('',(#4794,#4795,#4796,#4797));
#4992=CLOSED_SHELL('',(#4798));
#4993=CLOSED_SHELL('',(#4799));
#4994=CLOSED_SHELL('',(#4800,#4801,#4802,#4803,#4804,#4805,#4806,#4807));
#4995=CLOSED_SHELL('',(#4808,#4809,#4810,#4811,#4812,#4813,#4814,#4815));
#5298=AXIS2_PLACEMENT_3D('',#7823,#6258,#6259);
#5299=AXIS2_PLACEMENT_3D('',#7824,#6260,#6261);
#5300=AXIS2_PLACEMENT_3D('',#7826,#6262,#6263);
#5301=AXIS2_PLACEMENT_3D('',#7828,#6264,#6265);
#5302=AXIS2_PLACEMENT_3D('',#7829,#6266,#6267);
#5303=AXIS2_PLACEMENT_3D('',#7830,#6268,#6269);
#5304=AXIS2_PLACEMENT_3D('',#7832,#6270,#6271);
#5305=AXIS2_PLACEMENT_3D('',#7835,#6273,#6274);
#5306=AXIS2_PLACEMENT_3D('',#7836,#6275,#6276);
#5307=AXIS2_PLACEMENT_3D('',#7840,#6278,#6279);
#5308=AXIS2_PLACEMENT_3D('',#7841,#6280,#6281);
#5309=AXIS2_PLACEMENT_3D('',#7842,#6282,#6283);
#5310=AXIS2_PLACEMENT_3D('',#7845,#6285,#6286);
#5311=AXIS2_PLACEMENT_3D('',#7846,#6287,#6288);
#5312=AXIS2_PLACEMENT_3D('',#7848,#6289,#6290);
#5313=AXIS2_PLACEMENT_3D('',#7850,#6292,#6293);
#5314=AXIS2_PLACEMENT_3D('',#7853,#6295,#6296);
#5315=AXIS2_PLACEMENT_3D('',#7854,#6297,#6298);
#5316=AXIS2_PLACEMENT_3D('',#7855,#6299,#6300);
#5317=AXIS2_PLACEMENT_3D('',#7856,#6301,#6302);
#5318=AXIS2_PLACEMENT_3D('',#7859,#6303,#6304);
#5319=AXIS2_PLACEMENT_3D('',#7860,#6305,#6306);
#5320=AXIS2_PLACEMENT_3D('',#7862,#6307,#6308);
#5321=AXIS2_PLACEMENT_3D('',#7865,#6310,#6311);
#5322=AXIS2_PLACEMENT_3D('',#7866,#6312,#6313);
#5323=AXIS2_PLACEMENT_3D('',#7868,#6314,#6315);
#5324=AXIS2_PLACEMENT_3D('',#7871,#6317,#6318);
#5325=AXIS2_PLACEMENT_3D('',#7872,#6319,#6320);
#5326=AXIS2_PLACEMENT_3D('',#7874,#6321,#6322);
#5327=AXIS2_PLACEMENT_3D('',#7875,#6323,#6324);
#5328=AXIS2_PLACEMENT_3D('',#7876,#6325,#6326);
#5329=AXIS2_PLACEMENT_3D('',#7878,#6327,#6328);
#5330=AXIS2_PLACEMENT_3D('',#7880,#6330,#6331);
#5331=AXIS2_PLACEMENT_3D('',#7883,#6332,#6333);
#5332=AXIS2_PLACEMENT_3D('',#7884,#6334,#6335);
#5333=AXIS2_PLACEMENT_3D('',#7887,#6337,#6338);
#5334=AXIS2_PLACEMENT_3D('',#7888,#6339,#6340);
#5335=AXIS2_PLACEMENT_3D('',#7890,#6342,#6343);
#5336=AXIS2_PLACEMENT_3D('',#7891,#6344,#6345);
#5337=AXIS2_PLACEMENT_3D('',#7892,#6346,#6347);
#5338=AXIS2_PLACEMENT_3D('',#7895,#6348,#6349);
#5339=AXIS2_PLACEMENT_3D('',#7896,#6350,#6351);
#5340=AXIS2_PLACEMENT_3D('',#7899,#6352,#6353);
#5341=AXIS2_PLACEMENT_3D('',#7900,#6354,#6355);
#5342=AXIS2_PLACEMENT_3D('',#7903,#6356,#6357);
#5343=AXIS2_PLACEMENT_3D('',#7904,#6358,#6359);
#5344=AXIS2_PLACEMENT_3D('',#7907,#6360,#6361);
#5345=AXIS2_PLACEMENT_3D('',#7908,#6362,#6363);
#5346=AXIS2_PLACEMENT_3D('',#7911,#6364,#6365);
#5347=AXIS2_PLACEMENT_3D('',#7912,#6366,#6367);
#5348=AXIS2_PLACEMENT_3D('',#7915,#6368,#6369);
#5349=AXIS2_PLACEMENT_3D('',#7916,#6370,#6371);
#5350=AXIS2_PLACEMENT_3D('',#7919,#6372,#6373);
#5351=AXIS2_PLACEMENT_3D('',#7920,#6374,#6375);
#5352=AXIS2_PLACEMENT_3D('',#7923,#6376,#6377);
#5353=AXIS2_PLACEMENT_3D('',#7924,#6378,#6379);
#5354=AXIS2_PLACEMENT_3D('',#7927,#6380,#6381);
#5355=AXIS2_PLACEMENT_3D('',#7956,#6382,#6383);
#5356=AXIS2_PLACEMENT_3D('',#7958,#6384,#6385);
#5357=AXIS2_PLACEMENT_3D('',#7959,#6386,#6387);
#5358=AXIS2_PLACEMENT_3D('',#7960,#6388,#6389);
#5359=AXIS2_PLACEMENT_3D('',#7963,#6390,#6391);
#5360=AXIS2_PLACEMENT_3D('',#7965,#6392,#6393);
#5361=AXIS2_PLACEMENT_3D('',#7967,#6394,#6395);
#5362=AXIS2_PLACEMENT_3D('',#7968,#6396,#6397);
#5363=AXIS2_PLACEMENT_3D('',#7969,#6398,#6399);
#5364=AXIS2_PLACEMENT_3D('',#7998,#6400,#6401);
#5365=AXIS2_PLACEMENT_3D('',#8000,#6402,#6403);
#5366=AXIS2_PLACEMENT_3D('',#8001,#6404,#6405);
#5367=AXIS2_PLACEMENT_3D('',#8002,#6406,#6407);
#5368=AXIS2_PLACEMENT_3D('',#8005,#6408,#6409);
#5369=AXIS2_PLACEMENT_3D('',#8007,#6410,#6411);
#5370=AXIS2_PLACEMENT_3D('',#8009,#6412,#6413);
#5371=AXIS2_PLACEMENT_3D('',#8010,#6414,#6415);
#5372=AXIS2_PLACEMENT_3D('',#8011,#6416,#6417);
#5373=AXIS2_PLACEMENT_3D('',#8040,#6418,#6419);
#5374=AXIS2_PLACEMENT_3D('',#8042,#6420,#6421);
#5375=AXIS2_PLACEMENT_3D('',#8043,#6422,#6423);
#5376=AXIS2_PLACEMENT_3D('',#8044,#6424,#6425);
#5377=AXIS2_PLACEMENT_3D('',#8047,#6426,#6427);
#5378=AXIS2_PLACEMENT_3D('',#8049,#6428,#6429);
#5379=AXIS2_PLACEMENT_3D('',#8051,#6430,#6431);
#5380=AXIS2_PLACEMENT_3D('',#8052,#6432,#6433);
#5381=AXIS2_PLACEMENT_3D('',#8053,#6434,#6435);
#5382=AXIS2_PLACEMENT_3D('',#8082,#6436,#6437);
#5383=AXIS2_PLACEMENT_3D('',#8084,#6438,#6439);
#5384=AXIS2_PLACEMENT_3D('',#8085,#6440,#6441);
#5385=AXIS2_PLACEMENT_3D('',#8086,#6442,#6443);
#5386=AXIS2_PLACEMENT_3D('',#8089,#6444,#6445);
#5387=AXIS2_PLACEMENT_3D('',#8091,#6446,#6447);
#5388=AXIS2_PLACEMENT_3D('',#8093,#6448,#6449);
#5389=AXIS2_PLACEMENT_3D('',#8094,#6450,#6451);
#5390=AXIS2_PLACEMENT_3D('',#8095,#6452,#6453);
#5391=AXIS2_PLACEMENT_3D('',#8124,#6454,#6455);
#5392=AXIS2_PLACEMENT_3D('',#8126,#6456,#6457);
#5393=AXIS2_PLACEMENT_3D('',#8127,#6458,#6459);
#5394=AXIS2_PLACEMENT_3D('',#8128,#6460,#6461);
#5395=AXIS2_PLACEMENT_3D('',#8131,#6462,#6463);
#5396=AXIS2_PLACEMENT_3D('',#8133,#6464,#6465);
#5397=AXIS2_PLACEMENT_3D('',#8135,#6466,#6467);
#5398=AXIS2_PLACEMENT_3D('',#8136,#6468,#6469);
#5399=AXIS2_PLACEMENT_3D('',#8137,#6470,#6471);
#5400=AXIS2_PLACEMENT_3D('',#8166,#6472,#6473);
#5401=AXIS2_PLACEMENT_3D('',#8168,#6474,#6475);
#5402=AXIS2_PLACEMENT_3D('',#8169,#6476,#6477);
#5403=AXIS2_PLACEMENT_3D('',#8170,#6478,#6479);
#5404=AXIS2_PLACEMENT_3D('',#8173,#6480,#6481);
#5405=AXIS2_PLACEMENT_3D('',#8175,#6482,#6483);
#5406=AXIS2_PLACEMENT_3D('',#8177,#6484,#6485);
#5407=AXIS2_PLACEMENT_3D('',#8178,#6486,#6487);
#5408=AXIS2_PLACEMENT_3D('',#8179,#6488,#6489);
#5409=AXIS2_PLACEMENT_3D('',#8208,#6490,#6491);
#5410=AXIS2_PLACEMENT_3D('',#8210,#6492,#6493);
#5411=AXIS2_PLACEMENT_3D('',#8211,#6494,#6495);
#5412=AXIS2_PLACEMENT_3D('',#8212,#6496,#6497);
#5413=AXIS2_PLACEMENT_3D('',#8215,#6498,#6499);
#5414=AXIS2_PLACEMENT_3D('',#8217,#6500,#6501);
#5415=AXIS2_PLACEMENT_3D('',#8219,#6502,#6503);
#5416=AXIS2_PLACEMENT_3D('',#8220,#6504,#6505);
#5417=AXIS2_PLACEMENT_3D('',#8221,#6506,#6507);
#5418=AXIS2_PLACEMENT_3D('',#8250,#6508,#6509);
#5419=AXIS2_PLACEMENT_3D('',#8252,#6510,#6511);
#5420=AXIS2_PLACEMENT_3D('',#8253,#6512,#6513);
#5421=AXIS2_PLACEMENT_3D('',#8254,#6514,#6515);
#5422=AXIS2_PLACEMENT_3D('',#8257,#6516,#6517);
#5423=AXIS2_PLACEMENT_3D('',#8259,#6518,#6519);
#5424=AXIS2_PLACEMENT_3D('',#8261,#6520,#6521);
#5425=AXIS2_PLACEMENT_3D('',#8262,#6522,#6523);
#5426=AXIS2_PLACEMENT_3D('',#8263,#6524,#6525);
#5427=AXIS2_PLACEMENT_3D('',#8292,#6526,#6527);
#5428=AXIS2_PLACEMENT_3D('',#8294,#6528,#6529);
#5429=AXIS2_PLACEMENT_3D('',#8295,#6530,#6531);
#5430=AXIS2_PLACEMENT_3D('',#8296,#6532,#6533);
#5431=AXIS2_PLACEMENT_3D('',#8299,#6534,#6535);
#5432=AXIS2_PLACEMENT_3D('',#8301,#6536,#6537);
#5433=AXIS2_PLACEMENT_3D('',#8303,#6538,#6539);
#5434=AXIS2_PLACEMENT_3D('',#8304,#6540,#6541);
#5435=AXIS2_PLACEMENT_3D('',#8305,#6542,#6543);
#5436=AXIS2_PLACEMENT_3D('',#8334,#6544,#6545);
#5437=AXIS2_PLACEMENT_3D('',#8336,#6546,#6547);
#5438=AXIS2_PLACEMENT_3D('',#8337,#6548,#6549);
#5439=AXIS2_PLACEMENT_3D('',#8338,#6550,#6551);
#5440=AXIS2_PLACEMENT_3D('',#8341,#6552,#6553);
#5441=AXIS2_PLACEMENT_3D('',#8343,#6554,#6555);
#5442=AXIS2_PLACEMENT_3D('',#8345,#6556,#6557);
#5443=AXIS2_PLACEMENT_3D('',#8346,#6558,#6559);
#5444=AXIS2_PLACEMENT_3D('',#8347,#6560,#6561);
#5445=AXIS2_PLACEMENT_3D('',#8348,#6562,#6563);
#5446=AXIS2_PLACEMENT_3D('',#8350,#6564,#6565);
#5447=AXIS2_PLACEMENT_3D('',#8353,#6567,#6568);
#5448=AXIS2_PLACEMENT_3D('',#8354,#6569,#6570);
#5449=AXIS2_PLACEMENT_3D('',#8356,#6571,#6572);
#5450=AXIS2_PLACEMENT_3D('',#8359,#6574,#6575);
#5451=AXIS2_PLACEMENT_3D('',#8360,#6576,#6577);
#5452=AXIS2_PLACEMENT_3D('',#8361,#6578,#6579);
#5453=AXIS2_PLACEMENT_3D('',#8390,#6580,#6581);
#5454=AXIS2_PLACEMENT_3D('',#8392,#6582,#6583);
#5455=AXIS2_PLACEMENT_3D('',#8393,#6584,#6585);
#5456=AXIS2_PLACEMENT_3D('',#8394,#6586,#6587);
#5457=AXIS2_PLACEMENT_3D('',#8397,#6588,#6589);
#5458=AXIS2_PLACEMENT_3D('',#8399,#6590,#6591);
#5459=AXIS2_PLACEMENT_3D('',#8401,#6592,#6593);
#5460=AXIS2_PLACEMENT_3D('',#8402,#6594,#6595);
#5461=AXIS2_PLACEMENT_3D('',#8403,#6596,#6597);
#5462=AXIS2_PLACEMENT_3D('',#8432,#6598,#6599);
#5463=AXIS2_PLACEMENT_3D('',#8434,#6600,#6601);
#5464=AXIS2_PLACEMENT_3D('',#8435,#6602,#6603);
#5465=AXIS2_PLACEMENT_3D('',#8436,#6604,#6605);
#5466=AXIS2_PLACEMENT_3D('',#8439,#6606,#6607);
#5467=AXIS2_PLACEMENT_3D('',#8441,#6608,#6609);
#5468=AXIS2_PLACEMENT_3D('',#8443,#6610,#6611);
#5469=AXIS2_PLACEMENT_3D('',#8444,#6612,#6613);
#5470=AXIS2_PLACEMENT_3D('',#8445,#6614,#6615);
#5471=AXIS2_PLACEMENT_3D('',#8446,#6616,#6617);
#5472=AXIS2_PLACEMENT_3D('',#8449,#6618,#6619);
#5473=AXIS2_PLACEMENT_3D('',#8450,#6620,#6621);
#5474=AXIS2_PLACEMENT_3D('',#8453,#6622,#6623);
#5475=AXIS2_PLACEMENT_3D('',#8454,#6624,#6625);
#5476=AXIS2_PLACEMENT_3D('',#8456,#6626,#6627);
#5477=AXIS2_PLACEMENT_3D('',#8458,#6628,#6629);
#5478=AXIS2_PLACEMENT_3D('',#8460,#6630,#6631);
#5479=AXIS2_PLACEMENT_3D('',#8461,#6632,#6633);
#5480=AXIS2_PLACEMENT_3D('',#8462,#6634,#6635);
#5481=AXIS2_PLACEMENT_3D('',#8465,#6636,#6637);
#5482=AXIS2_PLACEMENT_3D('',#8467,#6638,#6639);
#5483=AXIS2_PLACEMENT_3D('',#8468,#6640,#6641);
#5484=AXIS2_PLACEMENT_3D('',#8469,#6642,#6643);
#5485=AXIS2_PLACEMENT_3D('',#8470,#6644,#6645);
#5486=AXIS2_PLACEMENT_3D('',#8473,#6646,#6647);
#5487=AXIS2_PLACEMENT_3D('',#8474,#6648,#6649);
#5488=AXIS2_PLACEMENT_3D('',#8476,#6651,#6652);
#5489=AXIS2_PLACEMENT_3D('',#8478,#6653,#6654);
#5490=AXIS2_PLACEMENT_3D('',#8480,#6656,#6657);
#5491=AXIS2_PLACEMENT_3D('',#8482,#6658,#6659);
#5492=AXIS2_PLACEMENT_3D('',#8485,#6661,#6662);
#5493=AXIS2_PLACEMENT_3D('',#8486,#6663,#6664);
#5494=AXIS2_PLACEMENT_3D('',#8488,#6666,#6667);
#5495=AXIS2_PLACEMENT_3D('',#8489,#6668,#6669);
#5496=AXIS2_PLACEMENT_3D('',#8490,#6670,#6671);
#5497=AXIS2_PLACEMENT_3D('',#8492,#6672,#6673);
#5498=AXIS2_PLACEMENT_3D('',#8494,#6674,#6675);
#5499=AXIS2_PLACEMENT_3D('',#8495,#6676,#6677);
#5500=AXIS2_PLACEMENT_3D('',#8496,#6678,#6679);
#5501=AXIS2_PLACEMENT_3D('',#8498,#6680,#6681);
#5502=AXIS2_PLACEMENT_3D('',#8500,#6682,#6683);
#5503=AXIS2_PLACEMENT_3D('',#8501,#6684,#6685);
#5504=AXIS2_PLACEMENT_3D('',#8502,#6686,#6687);
#5505=AXIS2_PLACEMENT_3D('',#8505,#6688,#6689);
#5506=AXIS2_PLACEMENT_3D('',#8506,#6690,#6691);
#5507=AXIS2_PLACEMENT_3D('',#8508,#6693,#6694);
#5508=AXIS2_PLACEMENT_3D('',#8510,#6695,#6696);
#5509=AXIS2_PLACEMENT_3D('',#8512,#6698,#6699);
#5510=AXIS2_PLACEMENT_3D('',#8514,#6700,#6701);
#5511=AXIS2_PLACEMENT_3D('',#8517,#6703,#6704);
#5512=AXIS2_PLACEMENT_3D('',#8518,#6705,#6706);
#5513=AXIS2_PLACEMENT_3D('',#8520,#6708,#6709);
#5514=AXIS2_PLACEMENT_3D('',#8521,#6710,#6711);
#6258=DIRECTION('axis',(0.,0.,1.));
#6259=DIRECTION('refdir',(1.,0.,0.));
#6260=DIRECTION('center_axis',(0.,-1.83697019872103E-16,-1.));
#6261=DIRECTION('ref_axis',(0.,-1.,1.83697019872103E-16));
#6262=DIRECTION('center_axis',(0.,1.83697019872103E-16,1.));
#6263=DIRECTION('ref_axis',(0.,-1.,1.83697019872103E-16));
#6264=DIRECTION('center_axis',(-1.,1.22464679914735E-16,-2.24963967399279E-32));
#6265=DIRECTION('ref_axis',(1.22464679914735E-16,1.,-1.83697019872103E-16));
#6266=DIRECTION('center_axis',(0.,1.83697019872103E-16,1.));
#6267=DIRECTION('ref_axis',(0.,-1.,1.83697019872103E-16));
#6268=DIRECTION('center_axis',(0.,-1.83697019872103E-16,-1.));
#6269=DIRECTION('ref_axis',(0.,-1.,1.83697019872103E-16));
#6270=DIRECTION('center_axis',(0.,1.83697019872103E-16,1.));
#6271=DIRECTION('ref_axis',(0.,-1.,1.83697019872103E-16));
#6272=DIRECTION('',(8.65956056235476E-17,0.707106781186533,-0.707106781186562));
#6273=DIRECTION('center_axis',(0.,1.83697019872103E-16,1.));
#6274=DIRECTION('ref_axis',(0.,-1.,1.83697019872103E-16));
#6275=DIRECTION('center_axis',(0.,1.83697019872103E-16,1.));
#6276=DIRECTION('ref_axis',(0.,-1.,1.83697019872103E-16));
#6277=DIRECTION('',(0.,1.83697019872103E-16,1.));
#6278=DIRECTION('center_axis',(0.,1.83697019872103E-16,1.));
#6279=DIRECTION('ref_axis',(0.,-1.,1.83697019872103E-16));
#6280=DIRECTION('center_axis',(0.,1.83697019872103E-16,1.));
#6281=DIRECTION('ref_axis',(0.,-1.,1.83697019872103E-16));
#6282=DIRECTION('center_axis',(0.,1.83697019872103E-16,1.));
#6283=DIRECTION('ref_axis',(0.,1.,-1.83697019872103E-16));
#6284=DIRECTION('',(8.65956056235476E-17,-0.707106781186533,0.707106781186562));
#6285=DIRECTION('center_axis',(0.,1.83697019872103E-16,1.));
#6286=DIRECTION('ref_axis',(0.,-1.,1.83697019872103E-16));
#6287=DIRECTION('center_axis',(0.,1.83697019872103E-16,1.));
#6288=DIRECTION('ref_axis',(0.,-1.,1.83697019872103E-16));
#6289=DIRECTION('center_axis',(0.,1.83697019872103E-16,1.));
#6290=DIRECTION('ref_axis',(0.,-1.,1.83697019872103E-16));
#6291=DIRECTION('',(0.,-1.83697019872103E-16,-1.));
#6292=DIRECTION('center_axis',(0.,1.83697019872103E-16,1.));
#6293=DIRECTION('ref_axis',(0.,-1.,1.83697019872103E-16));
#6294=DIRECTION('',(0.,-1.83697019872103E-16,-1.));
#6295=DIRECTION('center_axis',(0.,1.83697019872103E-16,1.));
#6296=DIRECTION('ref_axis',(0.,-1.,1.83697019872103E-16));
#6297=DIRECTION('center_axis',(0.,-1.83697019872103E-16,-1.));
#6298=DIRECTION('ref_axis',(0.,1.,-1.83697019872103E-16));
#6299=DIRECTION('center_axis',(0.,1.83697019872103E-16,1.));
#6300=DIRECTION('ref_axis',(0.,-1.,1.83697019872103E-16));
#6301=DIRECTION('center_axis',(-1.,0.,0.));
#6302=DIRECTION('ref_axis',(0.,1.,0.));
#6303=DIRECTION('center_axis',(0.,1.22464679914735E-16,1.));
#6304=DIRECTION('ref_axis',(0.,-1.,1.22464679914735E-16));
#6305=DIRECTION('center_axis',(0.,-1.83697019872103E-16,-1.));
#6306=DIRECTION('ref_axis',(0.,-1.,1.83697019872103E-16));
#6307=DIRECTION('center_axis',(0.,1.83697019872103E-16,1.));
#6308=DIRECTION('ref_axis',(0.,-1.,1.83697019872103E-16));
#6309=DIRECTION('',(-8.6595605623548E-17,-0.707106781186537,0.707106781186558));
#6310=DIRECTION('center_axis',(0.,1.83697019872103E-16,1.));
#6311=DIRECTION('ref_axis',(0.,-1.,1.83697019872103E-16));
#6312=DIRECTION('center_axis',(0.,1.83697019872103E-16,1.));
#6313=DIRECTION('ref_axis',(0.,-1.,1.83697019872103E-16));
#6314=DIRECTION('center_axis',(0.,1.83697019872103E-16,1.));
#6315=DIRECTION('ref_axis',(0.,-1.,1.83697019872103E-16));
#6316=DIRECTION('',(0.,1.83697019872103E-16,1.));
#6317=DIRECTION('center_axis',(0.,1.83697019872103E-16,1.));
#6318=DIRECTION('ref_axis',(0.,-1.,1.83697019872103E-16));
#6319=DIRECTION('center_axis',(0.,-1.83697019872103E-16,-1.));
#6320=DIRECTION('ref_axis',(0.,-1.,1.83697019872103E-16));
#6321=DIRECTION('center_axis',(-1.,1.22464679914735E-16,-2.24963967399279E-32));
#6322=DIRECTION('ref_axis',(1.22464679914735E-16,1.,-1.83697019872103E-16));
#6323=DIRECTION('center_axis',(0.,1.83697019872103E-16,1.));
#6324=DIRECTION('ref_axis',(0.,-1.,1.83697019872103E-16));
#6325=DIRECTION('center_axis',(0.,1.83697019872103E-16,1.));
#6326=DIRECTION('ref_axis',(0.,-1.,1.83697019872103E-16));
#6327=DIRECTION('center_axis',(0.,1.83697019872103E-16,1.));
#6328=DIRECTION('ref_axis',(0.,-1.,1.83697019872103E-16));
#6329=DIRECTION('',(0.,1.83697019872103E-16,1.));
#6330=DIRECTION('center_axis',(0.,1.83697019872103E-16,1.));
#6331=DIRECTION('ref_axis',(0.,1.,-1.83697019872103E-16));
#6332=DIRECTION('center_axis',(0.,1.83697019872103E-16,1.));
#6333=DIRECTION('ref_axis',(0.,-1.,1.83697019872103E-16));
#6334=DIRECTION('center_axis',(0.,1.83697019872103E-16,1.));
#6335=DIRECTION('ref_axis',(0.,-1.,1.83697019872103E-16));
#6336=DIRECTION('',(-8.6595605623548E-17,0.707106781186537,-0.707106781186558));
#6337=DIRECTION('center_axis',(0.,1.83697019872103E-16,1.));
#6338=DIRECTION('ref_axis',(0.,-1.,1.83697019872103E-16));
#6339=DIRECTION('center_axis',(0.,1.83697019872103E-16,1.));
#6340=DIRECTION('ref_axis',(0.,-1.,1.83697019872103E-16));
#6341=DIRECTION('',(0.,-1.83697019872103E-16,-1.));
#6342=DIRECTION('center_axis',(0.,-1.83697019872103E-16,-1.));
#6343=DIRECTION('ref_axis',(0.,1.,-1.83697019872103E-16));
#6344=DIRECTION('center_axis',(0.,1.83697019872103E-16,1.));
#6345=DIRECTION('ref_axis',(0.,-1.,1.83697019872103E-16));
#6346=DIRECTION('center_axis',(-0.866025403784438,0.500000000000001,-9.18485099360517E-17));
#6347=DIRECTION('ref_axis',(0.500000000000001,0.866025403784438,2.46107340633671E-17));
#6348=DIRECTION('center_axis',(-3.06161699786839E-17,1.30668257935858E-16,
1.));
#6349=DIRECTION('ref_axis',(-0.500000000000001,-0.866025403784438,9.78539458513683E-17));
#6350=DIRECTION('center_axis',(-0.499999999999998,0.86602540378444,-1.59086285808736E-16));
#6351=DIRECTION('ref_axis',(0.86602540378444,0.499999999999998,9.18485099360519E-17));
#6352=DIRECTION('center_axis',(-5.30287619362453E-17,1.53080849893419E-16,
1.));
#6353=DIRECTION('ref_axis',(-0.86602540378444,-0.499999999999998,3.06161699786834E-17));
#6354=DIRECTION('center_axis',(3.56496022900526E-15,1.,-1.83697019872103E-16));
#6355=DIRECTION('ref_axis',(1.,-3.56496022900527E-15,1.83697019872103E-16));
#6356=DIRECTION('center_axis',(-6.1232339957367E-17,1.83697019872103E-16,
1.));
#6357=DIRECTION('ref_axis',(-1.,3.56496022900527E-15,-6.12323399573677E-17));
#6358=DIRECTION('center_axis',(0.500000000000004,0.866025403784436,-1.59086285808735E-16));
#6359=DIRECTION('ref_axis',(0.866025403784436,-0.500000000000004,2.75545529808155E-16));
#6360=DIRECTION('center_axis',(-5.30287619362453E-17,2.14313189850786E-16,
1.));
#6361=DIRECTION('ref_axis',(-0.866025403784436,0.500000000000004,-1.5308084989342E-16));
#6362=DIRECTION('center_axis',(0.866025403784442,0.499999999999995,-9.18485099360505E-17));
#6363=DIRECTION('ref_axis',(0.499999999999995,-0.866025403784442,3.42783305680839E-16));
#6364=DIRECTION('center_axis',(-3.06161699786832E-17,2.36725781808348E-16,
1.));
#6365=DIRECTION('ref_axis',(-0.499999999999995,0.866025403784442,-2.20318625766104E-16));
#6366=DIRECTION('center_axis',(1.,0.,0.));
#6367=DIRECTION('ref_axis',(0.,-1.,3.67394039744206E-16));
#6368=DIRECTION('center_axis',(0.,2.44929359829471E-16,1.));
#6369=DIRECTION('ref_axis',(0.,1.,-2.44929359829471E-16));
#6370=DIRECTION('center_axis',(0.866025403784434,-0.500000000000008,9.18485099360529E-17));
#6371=DIRECTION('ref_axis',(-0.500000000000008,-0.866025403784434,3.42783305680838E-16));
#6372=DIRECTION('center_axis',(3.06161699786843E-17,2.36725781808348E-16,
1.));
#6373=DIRECTION('ref_axis',(0.500000000000008,0.866025403784434,-2.20318625766103E-16));
#6374=DIRECTION('center_axis',(0.499999999999992,-0.866025403784443,1.59086285808737E-16));
#6375=DIRECTION('ref_axis',(-0.866025403784443,-0.499999999999992,2.75545529808153E-16));
#6376=DIRECTION('center_axis',(5.30287619362456E-17,2.14313189850786E-16,
1.));
#6377=DIRECTION('ref_axis',(0.866025403784443,0.499999999999992,-1.53080849893418E-16));
#6378=DIRECTION('center_axis',(-1.06948806870158E-14,-1.,1.83697019872103E-16));
#6379=DIRECTION('ref_axis',(-1.,1.06948806870158E-14,1.83697019872101E-16));
#6380=DIRECTION('center_axis',(6.12323399573675E-17,1.83697019872102E-16,
1.));
#6381=DIRECTION('ref_axis',(1.,-1.06948806870158E-14,-6.12323399573656E-17));
#6382=DIRECTION('center_axis',(0.,-1.,0.));
#6383=DIRECTION('ref_axis',(0.,0.,-1.));
#6384=DIRECTION('center_axis',(-1.,2.84594884284774E-15,-1.22464679914694E-16));
#6385=DIRECTION('ref_axis',(-1.22464679914735E-16,-1.45251455301593E-14,
1.));
#6386=DIRECTION('center_axis',(0.,-1.,0.));
#6387=DIRECTION('ref_axis',(0.,0.,-1.));
#6388=DIRECTION('center_axis',(1.,0.,-1.22464679914735E-16));
#6389=DIRECTION('ref_axis',(-6.12323399573676E-17,0.,-1.));
#6390=DIRECTION('center_axis',(0.,1.,0.));
#6391=DIRECTION('ref_axis',(6.12323399573676E-17,0.,1.));
#6392=DIRECTION('center_axis',(0.,-1.,0.));
#6393=DIRECTION('ref_axis',(0.,0.,-1.));
#6394=DIRECTION('center_axis',(0.,-1.,0.));
#6395=DIRECTION('ref_axis',(0.,0.,-1.));
#6396=DIRECTION('center_axis',(0.,-1.,0.));
#6397=DIRECTION('ref_axis',(0.,0.,-1.));
#6398=DIRECTION('center_axis',(0.,1.,0.));
#6399=DIRECTION('ref_axis',(0.,0.,1.));
#6400=DIRECTION('center_axis',(-0.500000000000001,-0.866025403784438,-2.46107340633671E-17));
#6401=DIRECTION('ref_axis',(1.23053670316836E-17,2.13135209046589E-17,-1.));
#6402=DIRECTION('center_axis',(-0.866025403784473,0.49999999999994,-4.06043840956678E-14));
#6403=DIRECTION('ref_axis',(0.,8.12087681913454E-14,1.));
#6404=DIRECTION('center_axis',(-0.500000000000001,-0.866025403784438,-2.46107340633671E-17));
#6405=DIRECTION('ref_axis',(1.23053670316836E-17,2.13135209046589E-17,-1.));
#6406=DIRECTION('center_axis',(0.866025403784438,-0.500000000000001,-1.22464679914735E-16));
#6407=DIRECTION('ref_axis',(0.,0.,-1.));
#6408=DIRECTION('center_axis',(0.500000000000001,0.866025403784438,0.));
#6409=DIRECTION('ref_axis',(0.,0.,1.));
#6410=DIRECTION('center_axis',(-0.500000000000001,-0.866025403784438,-2.46107340633671E-17));
#6411=DIRECTION('ref_axis',(1.23053670316836E-17,2.13135209046589E-17,-1.));
#6412=DIRECTION('center_axis',(-0.500000000000001,-0.866025403784438,-2.46107340633671E-17));
#6413=DIRECTION('ref_axis',(1.23053670316836E-17,2.13135209046589E-17,-1.));
#6414=DIRECTION('center_axis',(-0.500000000000001,-0.866025403784438,-2.46107340633671E-17));
#6415=DIRECTION('ref_axis',(9.18485099360517E-17,-2.4610734063367E-17,-1.));
#6416=DIRECTION('center_axis',(0.500000000000001,0.866025403784438,2.46107340633671E-17));
#6417=DIRECTION('ref_axis',(-9.18485099360517E-17,2.4610734063367E-17,1.));
#6418=DIRECTION('center_axis',(-0.86602540378444,-0.499999999999998,-9.18485099360519E-17));
#6419=DIRECTION('ref_axis',(7.95431429043685E-17,4.59242549680258E-17,-1.));
#6420=DIRECTION('center_axis',(0.500000000000015,-0.86602540378443,-9.57339137215078E-15));
#6421=DIRECTION('ref_axis',(-1.9146782744301E-14,0.,-1.));
#6422=DIRECTION('center_axis',(-0.86602540378444,-0.499999999999998,-9.18485099360519E-17));
#6423=DIRECTION('ref_axis',(7.95431429043685E-17,4.59242549680258E-17,-1.));
#6424=DIRECTION('center_axis',(0.499999999999998,-0.86602540378444,-1.22464679914735E-16));
#6425=DIRECTION('ref_axis',(0.,0.,-1.));
#6426=DIRECTION('center_axis',(0.86602540378444,0.499999999999998,0.));
#6427=DIRECTION('ref_axis',(0.,0.,1.));
#6428=DIRECTION('center_axis',(-0.86602540378444,-0.499999999999998,-9.18485099360519E-17));
#6429=DIRECTION('ref_axis',(7.95431429043685E-17,4.59242549680257E-17,-1.));
#6430=DIRECTION('center_axis',(-0.86602540378444,-0.499999999999998,-9.18485099360519E-17));
#6431=DIRECTION('ref_axis',(7.95431429043685E-17,4.59242549680257E-17,-1.));
#6432=DIRECTION('center_axis',(-0.86602540378444,-0.499999999999998,-9.18485099360519E-17));
#6433=DIRECTION('ref_axis',(1.59086285808736E-16,-9.18485099360518E-17,
-1.));
#6434=DIRECTION('center_axis',(0.86602540378444,0.499999999999998,9.18485099360519E-17));
#6435=DIRECTION('ref_axis',(-1.59086285808736E-16,9.18485099360518E-17,
1.));
#6436=DIRECTION('center_axis',(-1.,3.49148133884313E-15,-1.83697019872104E-16));
#6437=DIRECTION('ref_axis',(1.83697019872103E-16,-1.83697019872105E-16,
-1.));
#6438=DIRECTION('center_axis',(-3.56732052431893E-15,-1.,1.22464679914626E-16));
#6439=DIRECTION('ref_axis',(3.03707588357877E-14,-1.22464679914735E-16,
-1.));
#6440=DIRECTION('center_axis',(-1.,3.49148133884313E-15,-1.83697019872104E-16));
#6441=DIRECTION('ref_axis',(1.83697019872103E-16,-1.83697019872105E-16,
-1.));
#6442=DIRECTION('center_axis',(-3.56496022900528E-15,-1.,6.12323399573673E-17));
#6443=DIRECTION('ref_axis',(0.,-1.22464679914736E-16,-1.));
#6444=DIRECTION('center_axis',(1.,-3.56496022900527E-15,4.36581713353893E-31));
#6445=DIRECTION('ref_axis',(0.,1.22464679914736E-16,1.));
#6446=DIRECTION('center_axis',(-1.,3.49148133884313E-15,-1.83697019872104E-16));
#6447=DIRECTION('ref_axis',(1.83697019872103E-16,-1.83697019872104E-16,
-1.));
#6448=DIRECTION('center_axis',(-1.,3.49148133884313E-15,-1.83697019872104E-16));
#6449=DIRECTION('ref_axis',(1.83697019872103E-16,-1.83697019872104E-16,
-1.));
#6450=DIRECTION('center_axis',(-1.,3.49148133884313E-15,-1.83697019872104E-16));
#6451=DIRECTION('ref_axis',(1.83697019872103E-16,-1.83697019872104E-16,
-1.));
#6452=DIRECTION('center_axis',(1.,-3.49148133884313E-15,1.83697019872104E-16));
#6453=DIRECTION('ref_axis',(-1.83697019872103E-16,1.83697019872104E-16,
1.));
#6454=DIRECTION('center_axis',(-0.866025403784436,0.500000000000004,-2.75545529808155E-16));
#6455=DIRECTION('ref_axis',(1.20569152228707E-16,-3.42259162130681E-16,
-1.));
#6456=DIRECTION('center_axis',(-0.499999999999989,-0.866025403784445,-2.60792385655128E-14));
#6457=DIRECTION('ref_axis',(5.21584771310268E-14,0.,-1.));
#6458=DIRECTION('center_axis',(-0.866025403784436,0.500000000000004,-2.75545529808155E-16));
#6459=DIRECTION('ref_axis',(2.5088757443104E-18,-5.46745559357283E-16,-1.));
#6460=DIRECTION('center_axis',(-0.500000000000004,-0.866025403784436,-1.22464679914735E-16));
#6461=DIRECTION('ref_axis',(0.,0.,-1.));
#6462=DIRECTION('center_axis',(0.866025403784436,-0.500000000000004,0.));
#6463=DIRECTION('ref_axis',(0.,0.,1.));
#6464=DIRECTION('center_axis',(-0.866025403784436,0.500000000000004,-2.75545529808155E-16));
#6465=DIRECTION('ref_axis',(1.05327043884768E-16,-3.68659268196852E-16,
-1.));
#6466=DIRECTION('center_axis',(-0.866025403784436,0.500000000000004,-2.75545529808155E-16));
#6467=DIRECTION('ref_axis',(2.38629428713104E-16,-1.37772764904079E-16,
-1.));
#6468=DIRECTION('center_axis',(-0.866025403784436,0.500000000000004,-2.75545529808155E-16));
#6469=DIRECTION('ref_axis',(1.59086285808736E-16,-2.75545529808155E-16,
-1.));
#6470=DIRECTION('center_axis',(0.866025403784436,-0.500000000000004,2.75545529808155E-16));
#6471=DIRECTION('ref_axis',(-1.59086285808736E-16,2.75545529808155E-16,
1.));
#6472=DIRECTION('center_axis',(-0.499999999999995,0.866025403784442,-3.4278330568084E-16));
#6473=DIRECTION('ref_axis',(-6.47289001283727E-17,-4.33183315530548E-16,
-1.));
#6474=DIRECTION('center_axis',(-0.866025403784424,-0.500000000000026,1.08638070651314E-13));
#6475=DIRECTION('ref_axis',(-1.25444438669558E-13,0.,-1.));
#6476=DIRECTION('center_axis',(-0.499999999999995,0.866025403784442,-3.4278330568084E-16));
#6477=DIRECTION('ref_axis',(-6.47289001283722E-17,-4.33183315530548E-16,
-1.));
#6478=DIRECTION('center_axis',(-0.866025403784442,-0.499999999999995,1.67652526221758E-16));
#6479=DIRECTION('ref_axis',(0.,-5.94160038167547E-16,-1.));
#6480=DIRECTION('center_axis',(0.499999999999995,-0.866025403784442,6.43197108708287E-16));
#6481=DIRECTION('ref_axis',(0.,7.42700047709434E-16,1.));
#6482=DIRECTION('center_axis',(-0.499999999999995,0.866025403784442,-3.4278330568084E-16));
#6483=DIRECTION('ref_axis',(-9.52131168162501E-17,-4.50783386241328E-16,
-1.));
#6484=DIRECTION('center_axis',(-0.499999999999995,0.866025403784442,-3.4278330568084E-16));
#6485=DIRECTION('ref_axis',(-9.52131168162501E-17,-4.50783386241328E-16,
-1.));
#6486=DIRECTION('center_axis',(-0.499999999999995,0.866025403784442,-3.4278330568084E-16));
#6487=DIRECTION('ref_axis',(9.18485099360505E-17,-3.4278330568084E-16,-1.));
#6488=DIRECTION('center_axis',(0.499999999999995,-0.866025403784442,3.4278330568084E-16));
#6489=DIRECTION('ref_axis',(-9.18485099360505E-17,3.4278330568084E-16,1.));
#6490=DIRECTION('center_axis',(0.,1.,-3.67394039744206E-16));
#6491=DIRECTION('ref_axis',(0.,-3.67394039744206E-16,-1.));
#6492=DIRECTION('center_axis',(-1.,-7.45578900633689E-15,1.22464679914593E-16));
#6493=DIRECTION('ref_axis',(-1.22464679914735E-16,1.91467827443009E-14,
-1.));
#6494=DIRECTION('center_axis',(0.,1.,-3.67394039744206E-16));
#6495=DIRECTION('ref_axis',(0.,-3.67394039744206E-16,-1.));
#6496=DIRECTION('center_axis',(-1.,0.,-1.22464679914735E-16));
#6497=DIRECTION('ref_axis',(6.12323399573676E-17,0.,-1.));
#6498=DIRECTION('center_axis',(0.,-1.,0.));
#6499=DIRECTION('ref_axis',(-6.12323399573676E-17,0.,1.));
#6500=DIRECTION('center_axis',(0.,1.,-3.67394039744206E-16));
#6501=DIRECTION('ref_axis',(0.,-3.67394039744206E-16,-1.));
#6502=DIRECTION('center_axis',(0.,1.,-3.67394039744206E-16));
#6503=DIRECTION('ref_axis',(0.,-3.67394039744206E-16,-1.));
#6504=DIRECTION('center_axis',(0.,1.,-3.67394039744206E-16));
#6505=DIRECTION('ref_axis',(0.,-3.67394039744206E-16,-1.));
#6506=DIRECTION('center_axis',(0.,-1.,3.67394039744206E-16));
#6507=DIRECTION('ref_axis',(0.,3.67394039744206E-16,1.));
#6508=DIRECTION('center_axis',(0.500000000000007,0.866025403784435,-3.42783305680838E-16));
#6509=DIRECTION('ref_axis',(6.47289001283733E-17,-4.3318331553055E-16,-1.));
#6510=DIRECTION('center_axis',(0.866025403784425,-0.500000000000023,4.66000145162218E-14));
#6511=DIRECTION('ref_axis',(-5.38090618503631E-14,0.,1.));
#6512=DIRECTION('center_axis',(0.500000000000007,0.866025403784435,-3.42783305680838E-16));
#6513=DIRECTION('ref_axis',(6.47289001283733E-17,-4.3318331553055E-16,-1.));
#6514=DIRECTION('center_axis',(-0.866025403784434,0.500000000000007,-4.12581886051237E-16));
#6515=DIRECTION('ref_axis',(0.,-5.94160038167547E-16,-1.));
#6516=DIRECTION('center_axis',(-0.500000000000007,-0.866025403784434,6.43197108708281E-16));
#6517=DIRECTION('ref_axis',(0.,7.42700047709434E-16,1.));
#6518=DIRECTION('center_axis',(0.500000000000007,0.866025403784435,-3.42783305680838E-16));
#6519=DIRECTION('ref_axis',(9.52131168162512E-17,-4.50783386241332E-16,
-1.));
#6520=DIRECTION('center_axis',(0.500000000000007,0.866025403784435,-3.42783305680838E-16));
#6521=DIRECTION('ref_axis',(9.52131168162512E-17,-4.50783386241332E-16,
-1.));
#6522=DIRECTION('center_axis',(0.500000000000007,0.866025403784435,-3.42783305680838E-16));
#6523=DIRECTION('ref_axis',(-9.18485099360527E-17,-3.42783305680838E-16,
-1.));
#6524=DIRECTION('center_axis',(-0.500000000000007,-0.866025403784435,3.42783305680838E-16));
#6525=DIRECTION('ref_axis',(9.18485099360527E-17,3.42783305680838E-16,1.));
#6526=DIRECTION('center_axis',(0.866025403784443,0.499999999999992,-2.75545529808153E-16));
#6527=DIRECTION('ref_axis',(-1.20569152228709E-16,-3.4225916213068E-16,
-1.));
#6528=DIRECTION('center_axis',(0.499999999999992,-0.866025403784443,-2.07973674636369E-14));
#6529=DIRECTION('ref_axis',(4.15947349272745E-14,0.,1.));
#6530=DIRECTION('center_axis',(0.866025403784443,0.499999999999992,-2.75545529808153E-16));
#6531=DIRECTION('ref_axis',(-2.5088757443144E-18,-5.46745559357285E-16,
-1.));
#6532=DIRECTION('center_axis',(-0.499999999999992,0.866025403784443,-1.22464679914735E-16));
#6533=DIRECTION('ref_axis',(0.,0.,-1.));
#6534=DIRECTION('center_axis',(-0.866025403784443,-0.499999999999992,0.));
#6535=DIRECTION('ref_axis',(0.,0.,1.));
#6536=DIRECTION('center_axis',(0.866025403784443,0.499999999999992,-2.75545529808153E-16));
#6537=DIRECTION('ref_axis',(-1.0532704388477E-16,-3.68659268196852E-16,
-1.));
#6538=DIRECTION('center_axis',(0.866025403784443,0.499999999999992,-2.75545529808153E-16));
#6539=DIRECTION('ref_axis',(-2.38629428713104E-16,-1.37772764904074E-16,
-1.));
#6540=DIRECTION('center_axis',(0.866025403784443,0.499999999999992,-2.75545529808153E-16));
#6541=DIRECTION('ref_axis',(-1.59086285808737E-16,-2.75545529808153E-16,
-1.));
#6542=DIRECTION('center_axis',(-0.866025403784443,-0.499999999999992,2.75545529808153E-16));
#6543=DIRECTION('ref_axis',(1.59086285808737E-16,2.75545529808153E-16,1.));
#6544=DIRECTION('center_axis',(1.,-1.04744440165294E-14,-1.83697019872101E-16));
#6545=DIRECTION('ref_axis',(-1.83697019872103E-16,-1.83697019872102E-16,
-1.));
#6546=DIRECTION('center_axis',(-3.12755891751053E-15,-1.,-1.22464679914974E-16));
#6547=DIRECTION('ref_axis',(-7.59268970894693E-14,-1.22464679914737E-16,
1.));
#6548=DIRECTION('center_axis',(1.,-1.04744440165294E-14,-1.83697019872101E-16));
#6549=DIRECTION('ref_axis',(-1.83697019872103E-16,-1.83697019872102E-16,
-1.));
#6550=DIRECTION('center_axis',(1.06948806870158E-14,1.,-3.06161699786834E-16));
#6551=DIRECTION('ref_axis',(0.,-2.44929359829463E-16,-1.));
#6552=DIRECTION('center_axis',(-1.,1.06948806870158E-14,-2.61949028012324E-30));
#6553=DIRECTION('ref_axis',(0.,2.44929359829461E-16,1.));
#6554=DIRECTION('center_axis',(1.,-1.04744440165294E-14,-1.83697019872101E-16));
#6555=DIRECTION('ref_axis',(-1.83697019872103E-16,-1.83697019872101E-16,
-1.));
#6556=DIRECTION('center_axis',(1.,-1.04744440165294E-14,-1.83697019872101E-16));
#6557=DIRECTION('ref_axis',(-1.83697019872103E-16,-1.83697019872101E-16,
-1.));
#6558=DIRECTION('center_axis',(1.,-1.04744440165294E-14,-1.83697019872101E-16));
#6559=DIRECTION('ref_axis',(-1.83697019872103E-16,-1.83697019872101E-16,
-1.));
#6560=DIRECTION('center_axis',(-1.,1.04744440165294E-14,1.83697019872101E-16));
#6561=DIRECTION('ref_axis',(1.83697019872103E-16,1.83697019872101E-16,1.));
#6562=DIRECTION('center_axis',(0.,0.,-1.));
#6563=DIRECTION('ref_axis',(-1.,0.,0.));
#6564=DIRECTION('center_axis',(0.,0.,1.));
#6565=DIRECTION('ref_axis',(1.,0.,0.));
#6566=DIRECTION('',(0.,0.,-1.));
#6567=DIRECTION('center_axis',(0.,0.,1.));
#6568=DIRECTION('ref_axis',(1.,0.,0.));
#6569=DIRECTION('center_axis',(0.,0.,-1.));
#6570=DIRECTION('ref_axis',(-1.,0.,0.));
#6571=DIRECTION('center_axis',(0.,0.,1.));
#6572=DIRECTION('ref_axis',(1.,0.,0.));
#6573=DIRECTION('',(0.,0.,1.));
#6574=DIRECTION('center_axis',(0.,0.,1.));
#6575=DIRECTION('ref_axis',(1.,0.,0.));
#6576=DIRECTION('center_axis',(0.,0.,1.));
#6577=DIRECTION('ref_axis',(1.,0.,0.));
#6578=DIRECTION('center_axis',(0.,0.,1.));
#6579=DIRECTION('ref_axis',(1.,0.,0.));
#6580=DIRECTION('center_axis',(0.866025403784433,-0.50000000000001,-9.18485099360496E-17));
#6581=DIRECTION('ref_axis',(-7.95431429043658E-17,4.59242549680257E-17,
-1.));
#6582=DIRECTION('center_axis',(-0.499999999999991,-0.866025403784444,-6.60233887734503E-16));
#6583=DIRECTION('ref_axis',(-1.32046777546903E-15,0.,1.));
#6584=DIRECTION('center_axis',(0.866025403784433,-0.50000000000001,-9.18485099360496E-17));
#6585=DIRECTION('ref_axis',(-7.95431429043658E-17,4.59242549680257E-17,
-1.));
#6586=DIRECTION('center_axis',(0.50000000000001,0.866025403784433,-1.22464679914735E-16));
#6587=DIRECTION('ref_axis',(0.,0.,-1.));
#6588=DIRECTION('center_axis',(-0.866025403784433,0.50000000000001,0.));
#6589=DIRECTION('ref_axis',(0.,0.,1.));
#6590=DIRECTION('center_axis',(0.866025403784433,-0.50000000000001,-9.18485099360496E-17));
#6591=DIRECTION('ref_axis',(-7.95431429043658E-17,4.59242549680257E-17,
-1.));
#6592=DIRECTION('center_axis',(0.866025403784433,-0.50000000000001,-9.18485099360496E-17));
#6593=DIRECTION('ref_axis',(-7.95431429043658E-17,4.59242549680257E-17,
-1.));
#6594=DIRECTION('center_axis',(0.866025403784433,-0.50000000000001,-9.18485099360497E-17));
#6595=DIRECTION('ref_axis',(-1.59086285808735E-16,-9.18485099360497E-17,
-1.));
#6596=DIRECTION('center_axis',(-0.866025403784433,0.50000000000001,9.18485099360497E-17));
#6597=DIRECTION('ref_axis',(1.59086285808735E-16,9.18485099360497E-17,1.));
#6598=DIRECTION('center_axis',(0.499999999999989,-0.866025403784445,-2.46107340633658E-17));
#6599=DIRECTION('ref_axis',(-1.23053670316826E-17,2.1313520904658E-17,-1.));
#6600=DIRECTION('center_axis',(-0.866025403784448,-0.499999999999983,-1.32046777546899E-15));
#6601=DIRECTION('ref_axis',(0.,-2.64093555093807E-15,1.));
#6602=DIRECTION('center_axis',(0.499999999999989,-0.866025403784445,-2.46107340633658E-17));
#6603=DIRECTION('ref_axis',(-1.23053670316826E-17,2.1313520904658E-17,-1.));
#6604=DIRECTION('center_axis',(0.866025403784445,0.499999999999989,-1.22464679914735E-16));
#6605=DIRECTION('ref_axis',(0.,0.,-1.));
#6606=DIRECTION('center_axis',(-0.499999999999989,0.866025403784445,0.));
#6607=DIRECTION('ref_axis',(0.,0.,1.));
#6608=DIRECTION('center_axis',(0.499999999999989,-0.866025403784445,-2.46107340633658E-17));
#6609=DIRECTION('ref_axis',(-1.23053670316826E-17,2.1313520904658E-17,-1.));
#6610=DIRECTION('center_axis',(0.499999999999989,-0.866025403784445,-2.46107340633658E-17));
#6611=DIRECTION('ref_axis',(-1.23053670316826E-17,2.1313520904658E-17,-1.));
#6612=DIRECTION('center_axis',(0.499999999999989,-0.866025403784445,-2.46107340633658E-17));
#6613=DIRECTION('ref_axis',(-9.18485099360495E-17,-2.46107340633658E-17,
-1.));
#6614=DIRECTION('center_axis',(-0.499999999999989,0.866025403784445,2.46107340633658E-17));
#6615=DIRECTION('ref_axis',(9.18485099360495E-17,2.46107340633658E-17,1.));
#6616=DIRECTION('center_axis',(-0.50000000000001,-0.866025403784433,1.59086285808735E-16));
#6617=DIRECTION('ref_axis',(-0.866025403784433,0.50000000000001,9.18485099360498E-17));
#6618=DIRECTION('center_axis',(5.30287619362451E-17,1.53080849893418E-16,
1.));
#6619=DIRECTION('ref_axis',(0.866025403784433,-0.50000000000001,3.06161699786855E-17));
#6620=DIRECTION('center_axis',(-0.866025403784446,-0.499999999999988,9.18485099360495E-17));
#6621=DIRECTION('ref_axis',(-0.499999999999988,0.866025403784445,2.46107340633657E-17));
#6622=DIRECTION('center_axis',(3.06161699786833E-17,1.30668257935857E-16,
1.));
#6623=DIRECTION('ref_axis',(0.499999999999988,-0.866025403784445,9.78539458513696E-17));
#6624=DIRECTION('center_axis',(0.,1.83697019872103E-16,1.));
#6625=DIRECTION('ref_axis',(0.,1.,-1.78694614991829E-16));
#6626=DIRECTION('center_axis',(0.,-1.83697019872103E-16,-1.));
#6627=DIRECTION('ref_axis',(0.,1.,-1.83697019872103E-16));
#6628=DIRECTION('center_axis',(1.,1.22464679914735E-16,-2.24963967399279E-32));
#6629=DIRECTION('ref_axis',(1.22464679914735E-16,-1.,1.86140223949822E-16));
#6630=DIRECTION('center_axis',(0.,1.83697019872103E-16,1.));
#6631=DIRECTION('ref_axis',(0.,1.,-1.83697019872103E-16));
#6632=DIRECTION('center_axis',(0.,1.83697019872103E-16,1.));
#6633=DIRECTION('ref_axis',(0.,1.,-1.83697019872103E-16));
#6634=DIRECTION('center_axis',(0.,1.83697019872103E-16,1.));
#6635=DIRECTION('ref_axis',(0.,1.,-1.95204048285742E-16));
#6636=DIRECTION('center_axis',(0.,-1.83697019872103E-16,-1.));
#6637=DIRECTION('ref_axis',(0.,1.,-1.83697019872103E-16));
#6638=DIRECTION('center_axis',(1.,1.22464679914735E-16,-2.24963967399279E-32));
#6639=DIRECTION('ref_axis',(1.22464679914735E-16,-1.,1.83003795267883E-16));
#6640=DIRECTION('center_axis',(0.,1.83697019872103E-16,1.));
#6641=DIRECTION('ref_axis',(0.,1.,-1.83697019872103E-16));
#6642=DIRECTION('center_axis',(0.,-1.83697019872103E-16,-1.));
#6643=DIRECTION('ref_axis',(0.,1.,-1.83697019872103E-16));
#6644=DIRECTION('center_axis',(0.,1.83697019872103E-16,1.));
#6645=DIRECTION('ref_axis',(0.,-1.,1.83697019872103E-16));
#6646=DIRECTION('center_axis',(0.,1.83697019872103E-16,1.));
#6647=DIRECTION('ref_axis',(0.,-1.,1.83697019872103E-16));
#6648=DIRECTION('center_axis',(0.,1.83697019872103E-16,1.));
#6649=DIRECTION('ref_axis',(0.,-1.,1.83697019872103E-16));
#6650=DIRECTION('',(0.,-1.83697019872103E-16,-1.));
#6651=DIRECTION('center_axis',(0.,1.83697019872103E-16,1.));
#6652=DIRECTION('ref_axis',(0.,1.,-1.83697019872103E-16));
#6653=DIRECTION('center_axis',(0.,1.83697019872103E-16,1.));
#6654=DIRECTION('ref_axis',(0.,-1.,1.83697019872103E-16));
#6655=DIRECTION('',(-1.0420961835668E-16,0.850936110144042,-0.525269203792614));
#6656=DIRECTION('center_axis',(0.,-1.83697019872103E-16,-1.));
#6657=DIRECTION('ref_axis',(0.,-1.,1.83697019872103E-16));
#6658=DIRECTION('center_axis',(0.,1.83697019872103E-16,1.));
#6659=DIRECTION('ref_axis',(0.,-1.,1.83697019872103E-16));
#6660=DIRECTION('',(1.0420961835668E-16,0.850936110144042,-0.525269203792614));
#6661=DIRECTION('center_axis',(0.,1.83697019872103E-16,1.));
#6662=DIRECTION('ref_axis',(0.,-1.,1.83697019872103E-16));
#6663=DIRECTION('center_axis',(0.,1.83697019872103E-16,1.));
#6664=DIRECTION('ref_axis',(0.,-1.,1.83697019872103E-16));
#6665=DIRECTION('',(0.,1.83697019872103E-16,1.));
#6666=DIRECTION('center_axis',(0.,-1.83697019872103E-16,-1.));
#6667=DIRECTION('ref_axis',(0.,1.,-1.83697019872103E-16));
#6668=DIRECTION('center_axis',(0.,1.83697019872103E-16,1.));
#6669=DIRECTION('ref_axis',(0.,-1.,1.83697019872103E-16));
#6670=DIRECTION('center_axis',(0.,-1.83697019872103E-16,-1.));
#6671=DIRECTION('ref_axis',(0.,-1.,1.95204048285742E-16));
#6672=DIRECTION('center_axis',(0.,1.83697019872103E-16,1.));
#6673=DIRECTION('ref_axis',(0.,-1.,1.83697019872103E-16));
#6674=DIRECTION('center_axis',(1.,-1.22464679914735E-16,2.24963967399279E-32));
#6675=DIRECTION('ref_axis',(1.22464679914735E-16,1.,-1.83003795267883E-16));
#6676=DIRECTION('center_axis',(0.,-1.83697019872103E-16,-1.));
#6677=DIRECTION('ref_axis',(0.,-1.,1.83697019872103E-16));
#6678=DIRECTION('center_axis',(0.,-1.83697019872103E-16,-1.));
#6679=DIRECTION('ref_axis',(0.,-1.,1.78694614991829E-16));
#6680=DIRECTION('center_axis',(0.,1.83697019872103E-16,1.));
#6681=DIRECTION('ref_axis',(0.,-1.,1.83697019872103E-16));
#6682=DIRECTION('center_axis',(1.,-1.22464679914735E-16,2.24963967399279E-32));
#6683=DIRECTION('ref_axis',(1.22464679914735E-16,1.,-1.86140223949822E-16));
#6684=DIRECTION('center_axis',(0.,-1.83697019872103E-16,-1.));
#6685=DIRECTION('ref_axis',(0.,-1.,1.83697019872103E-16));
#6686=DIRECTION('center_axis',(0.,1.83697019872103E-16,1.));
#6687=DIRECTION('ref_axis',(0.,-1.,1.83697019872103E-16));
#6688=DIRECTION('center_axis',(0.,1.83697019872103E-16,1.));
#6689=DIRECTION('ref_axis',(0.,-1.,1.83697019872103E-16));
#6690=DIRECTION('center_axis',(0.,1.83697019872103E-16,1.));
#6691=DIRECTION('ref_axis',(0.,-1.,1.83697019872103E-16));
#6692=DIRECTION('',(0.,1.83697019872103E-16,1.));
#6693=DIRECTION('center_axis',(0.,1.83697019872103E-16,1.));
#6694=DIRECTION('ref_axis',(0.,1.,-1.83697019872103E-16));
#6695=DIRECTION('center_axis',(0.,1.83697019872103E-16,1.));
#6696=DIRECTION('ref_axis',(0.,-1.,1.83697019872103E-16));
#6697=DIRECTION('',(1.0420961835668E-16,-0.850936110144042,0.525269203792614));
#6698=DIRECTION('center_axis',(0.,-1.83697019872103E-16,-1.));
#6699=DIRECTION('ref_axis',(0.,-1.,1.83697019872103E-16));
#6700=DIRECTION('center_axis',(0.,1.83697019872103E-16,1.));
#6701=DIRECTION('ref_axis',(0.,-1.,1.83697019872103E-16));
#6702=DIRECTION('',(-1.0420961835668E-16,-0.850936110144042,0.525269203792614));
#6703=DIRECTION('center_axis',(0.,1.83697019872103E-16,1.));
#6704=DIRECTION('ref_axis',(0.,-1.,1.83697019872103E-16));
#6705=DIRECTION('center_axis',(0.,1.83697019872103E-16,1.));
#6706=DIRECTION('ref_axis',(0.,-1.,1.83697019872103E-16));
#6707=DIRECTION('',(0.,-1.83697019872103E-16,-1.));
#6708=DIRECTION('center_axis',(0.,-1.83697019872103E-16,-1.));
#6709=DIRECTION('ref_axis',(0.,1.,-1.83697019872103E-16));
#6710=DIRECTION('center_axis',(0.,1.83697019872103E-16,1.));
#6711=DIRECTION('ref_axis',(0.,-1.,1.83697019872103E-16));
#7823=CARTESIAN_POINT('',(0.,0.,0.));
#7824=CARTESIAN_POINT('Origin',(0.,0.,1.30104260698261E-15));
#7825=CARTESIAN_POINT('',(8.8786892938183E-16,7.24999999999999,-1.11111111111111));
#7826=CARTESIAN_POINT('Origin',(0.,2.55134749822366E-16,-1.11111111111111));
#7827=CARTESIAN_POINT('',(-8.8786892938183E-16,7.24999999999999,1.11111111111111));
#7828=CARTESIAN_POINT('Origin',(1.01033360929657E-15,8.25,-2.1445780696224E-16));
#7829=CARTESIAN_POINT('Origin',(0.,6.6335034953815E-16,1.11111111111111));
#7830=CARTESIAN_POINT('Origin',(0.,-4.26423346241407E-31,-2.5));
#7831=CARTESIAN_POINT('',(-7.34788079488412E-16,6.,-2.25000000000001));
#7832=CARTESIAN_POINT('Origin',(0.,4.5924254968025E-17,-2.25));
#7833=CARTESIAN_POINT('',(-7.65404249467094E-16,6.24999999999999,-2.5));
#7834=CARTESIAN_POINT('',(7.65404249467095E-16,6.24999999999999,-2.5));
#7835=CARTESIAN_POINT('Origin',(0.,-4.26423346241407E-31,-2.5));
#7836=CARTESIAN_POINT('Origin',(0.,0.,-2.5));
#7837=CARTESIAN_POINT('',(-7.34788079488412E-16,6.,2.25000000000001));
#7838=CARTESIAN_POINT('',(-7.34788079488412E-16,6.,-2.5));
#7839=CARTESIAN_POINT('',(7.50096164477753E-16,-6.,2.25000000000001));
#7840=CARTESIAN_POINT('Origin',(0.,8.7256084439249E-16,2.25000000000001));
#7841=CARTESIAN_POINT('Origin',(0.,8.7256084439249E-16,2.25000000000001));
#7842=CARTESIAN_POINT('Origin',(0.,8.7256084439249E-16,2.25000000000001));
#7843=CARTESIAN_POINT('',(-7.65404249467094E-16,-6.24999999999999,2.50000000000001));
#7844=CARTESIAN_POINT('',(7.34788079488412E-16,-6.,2.25000000000001));
#7845=CARTESIAN_POINT('Origin',(0.,9.18485099360516E-16,2.5));
#7846=CARTESIAN_POINT('Origin',(0.,0.,-2.5));
#7847=CARTESIAN_POINT('',(-8.8786892938183E-16,7.24999999999999,2.5));
#7848=CARTESIAN_POINT('Origin',(0.,9.18485099360516E-16,2.50000000000001));
#7849=CARTESIAN_POINT('',(-8.8786892938183E-16,7.24999999999999,-2.5));
#7850=CARTESIAN_POINT('Origin',(0.,0.,-2.5));
#7851=CARTESIAN_POINT('',(-8.8786892938183E-16,7.24999999999999,-2.5));
#7852=CARTESIAN_POINT('',(-8.8786892938183E-16,7.24999999999999,-2.5));
#7853=CARTESIAN_POINT('Origin',(0.,-3.92678751131515E-31,-2.5));
#7854=CARTESIAN_POINT('Origin',(0.,6.24999999999999,-2.5));
#7855=CARTESIAN_POINT('Origin',(0.,6.24999999999999,2.5));
#7856=CARTESIAN_POINT('Origin',(0.,8.25,0.));
#7857=CARTESIAN_POINT('',(-1.49484711634153,8.25,1.12095579315854E-32));
#7858=CARTESIAN_POINT('',(1.49484711634153,8.25,1.12095579315854E-32));
#7859=CARTESIAN_POINT('Origin',(0.,8.25,0.));
#7860=CARTESIAN_POINT('Origin',(0.,9.18485099360516E-16,2.5));
#7861=CARTESIAN_POINT('',(-1.28587913910472E-15,10.5,2.25000000000001));
#7862=CARTESIAN_POINT('Origin',(0.,8.72560844392491E-16,2.25000000000001));
#7863=CARTESIAN_POINT('',(-1.25526296912604E-15,10.25,2.5));
#7864=CARTESIAN_POINT('',(1.25526296912604E-15,10.25,2.5));
#7865=CARTESIAN_POINT('Origin',(0.,9.18485099360516E-16,2.5));
#7866=CARTESIAN_POINT('Origin',(0.,0.,-2.5));
#7867=CARTESIAN_POINT('',(-1.1327982892113E-15,9.25000000000001,1.11111111111111));
#7868=CARTESIAN_POINT('Origin',(0.,6.6335034953815E-16,1.11111111111111));
#7869=CARTESIAN_POINT('',(-1.1327982892113E-15,9.25000000000001,2.50000000000001));
#7870=CARTESIAN_POINT('',(-1.1327982892113E-15,9.25000000000001,-2.5));
#7871=CARTESIAN_POINT('Origin',(0.,9.18485099360517E-16,2.50000000000001));
#7872=CARTESIAN_POINT('Origin',(0.,0.,1.30104260698261E-15));
#7873=CARTESIAN_POINT('',(-1.1327982892113E-15,9.25,-1.11111111111111));
#7874=CARTESIAN_POINT('Origin',(1.01033360929657E-15,8.25,-2.1445780696224E-16));
#7875=CARTESIAN_POINT('Origin',(0.,2.55134749822365E-16,-1.11111111111111));
#7876=CARTESIAN_POINT('Origin',(0.,0.,-2.5));
#7877=CARTESIAN_POINT('',(-1.1327982892113E-15,9.25,-2.5));
#7878=CARTESIAN_POINT('Origin',(0.,6.30801037605615E-31,-2.5));
#7879=CARTESIAN_POINT('',(-1.1327982892113E-15,9.25,-2.5));
#7880=CARTESIAN_POINT('Origin',(0.,4.59242549680263E-17,-2.25));
#7881=CARTESIAN_POINT('',(1.28587913910472E-15,10.5,-2.25));
#7882=CARTESIAN_POINT('',(1.28587913910472E-15,-10.5,-2.25));
#7883=CARTESIAN_POINT('Origin',(0.,4.59242549680263E-17,-2.25));
#7884=CARTESIAN_POINT('Origin',(0.,4.59242549680263E-17,-2.25));
#7885=CARTESIAN_POINT('',(-1.25526296912604E-15,-10.25,-2.49999999999999));
#7886=CARTESIAN_POINT('',(1.28587913910472E-15,-10.5,-2.25));
#7887=CARTESIAN_POINT('Origin',(0.,9.83209165554622E-31,-2.5));
#7888=CARTESIAN_POINT('Origin',(0.,0.,-2.5));
#7889=CARTESIAN_POINT('',(-1.28587913910472E-15,10.5,-2.5));
#7890=CARTESIAN_POINT('Origin',(0.,10.25,-2.5));
#7891=CARTESIAN_POINT('Origin',(0.,10.25,2.5));
#7892=CARTESIAN_POINT('Origin',(4.12500000000001,7.14470958122162,2.03038556022778E-16));
#7893=CARTESIAN_POINT('',(2.83042442247433,7.89213313939239,6.57390758046047E-17));
#7894=CARTESIAN_POINT('',(5.41957557752569,6.39728602305085,3.40338036240951E-16));
#7895=CARTESIAN_POINT('Origin',(4.12500000000001,7.14470958122162,2.03038556022778E-16));
#7896=CARTESIAN_POINT('Origin',(7.14470958122163,4.12499999999998,7.57750206972428E-16));
#7897=CARTESIAN_POINT('',(6.39728602305087,5.41957557752566,5.19940531381754E-16));
#7898=CARTESIAN_POINT('',(7.89213313939239,2.8304244224743,9.95559882563102E-16));
#7899=CARTESIAN_POINT('Origin',(7.14470958122163,4.12499999999998,7.57750206972428E-16));
#7900=CARTESIAN_POINT('Origin',(8.25,-2.88047210454559E-14,1.51550041394486E-15));
#7901=CARTESIAN_POINT('',(8.25000000000001,1.4948471163415,1.24090145350851E-15));
#7902=CARTESIAN_POINT('',(8.24999999999999,-1.49484711634156,1.79009937438121E-15));
#7903=CARTESIAN_POINT('Origin',(8.25,-2.88047210454559E-14,1.51550041394486E-15));
#7904=CARTESIAN_POINT('Origin',(7.1447095812216,-4.12500000000003,2.27325062091728E-15));
#7905=CARTESIAN_POINT('',(7.89213313939237,-2.83042442247436,2.03544094532661E-15));
#7906=CARTESIAN_POINT('',(6.39728602305083,-5.4195755775257,2.51106029650795E-15));
#7907=CARTESIAN_POINT('Origin',(7.1447095812216,-4.12500000000003,2.27325062091728E-15));
#7908=CARTESIAN_POINT('Origin',(4.12499999999996,-7.14470958122164,2.82796227186693E-15));
#7909=CARTESIAN_POINT('',(5.41957557752564,-6.39728602305088,2.69066279164876E-15));
#7910=CARTESIAN_POINT('',(2.83042442247428,-7.8921331393924,2.9652617520851E-15));
#7911=CARTESIAN_POINT('Origin',(4.12499999999996,-7.14470958122164,2.82796227186693E-15));
#7912=CARTESIAN_POINT('Origin',(0.,-8.25,3.0310008278897E-15));
#7913=CARTESIAN_POINT('',(1.49484711634153,-8.25,3.0310008278897E-15));
#7914=CARTESIAN_POINT('',(-1.49484711634153,-8.25,3.0310008278897E-15));
#7915=CARTESIAN_POINT('Origin',(0.,-8.25,3.0310008278897E-15));
#7916=CARTESIAN_POINT('Origin',(-4.12500000000006,-7.14470958122159,2.82796227186692E-15));
#7917=CARTESIAN_POINT('',(-2.83042442247439,-7.89213313939237,2.9652617520851E-15));
#7918=CARTESIAN_POINT('',(-5.41957557752573,-6.39728602305081,2.69066279164875E-15));
#7919=CARTESIAN_POINT('Origin',(-4.12500000000006,-7.14470958122159,2.82796227186692E-15));
#7920=CARTESIAN_POINT('Origin',(-7.14470958122166,-4.12499999999993,2.27325062091726E-15));
#7921=CARTESIAN_POINT('',(-6.39728602305091,-5.41957557752561,2.51106029650794E-15));
#7922=CARTESIAN_POINT('',(-7.89213313939241,-2.83042442247425,2.03544094532659E-15));
#7923=CARTESIAN_POINT('Origin',(-7.14470958122166,-4.12499999999993,2.27325062091726E-15));
#7924=CARTESIAN_POINT('Origin',(-8.25,8.64141631363676E-14,1.51550041394483E-15));
#7925=CARTESIAN_POINT('',(-8.25000000000002,-1.49484711634144,1.79009937438118E-15));
#7926=CARTESIAN_POINT('',(-8.24999999999999,1.49484711634162,1.24090145350848E-15));
#7927=CARTESIAN_POINT('Origin',(-8.25,8.64141631363676E-14,1.51550041394483E-15));
#7928=CARTESIAN_POINT('Ctrl Pts',(1.43761115075249E-15,8.75,1.59062243825056));
#7929=CARTESIAN_POINT('Ctrl Pts',(-1.59062243825055,8.75000000000001,1.59062243825056));
#7930=CARTESIAN_POINT('Ctrl Pts',(-1.59062243825055,8.75000000000003,6.65240462528331E-15));
#7931=CARTESIAN_POINT('Ctrl Pts',(-1.59062243825055,8.75000000000005,-1.59062243825054));
#7932=CARTESIAN_POINT('Ctrl Pts',(1.43761115075249E-15,8.75000000000005,
-1.59062243825054));
#7933=CARTESIAN_POINT('Ctrl Pts',(1.59062243825055,8.75000000000004,-1.59062243825054));
#7934=CARTESIAN_POINT('Ctrl Pts',(1.59062243825055,8.75000000000002,6.65240462528319E-15));
#7935=CARTESIAN_POINT('Ctrl Pts',(1.59062243825055,8.75,1.59062243825056));
#7936=CARTESIAN_POINT('Ctrl Pts',(1.43761115075249E-15,8.75,1.59062243825056));
#7937=CARTESIAN_POINT('Ctrl Pts',(1.46367293285559E-17,8.24999999999998,
1.77871997289447));
#7938=CARTESIAN_POINT('Ctrl Pts',(-1.77871997289447,8.24999999999998,1.77871997289447));
#7939=CARTESIAN_POINT('Ctrl Pts',(-1.77871997289447,8.25000000000001,-4.8572257327343E-16));
#7940=CARTESIAN_POINT('Ctrl Pts',(-1.77871997289447,8.25000000000003,-1.77871997289447));
#7941=CARTESIAN_POINT('Ctrl Pts',(1.46367293285536E-17,8.25000000000003,
-1.77871997289447));
#7942=CARTESIAN_POINT('Ctrl Pts',(1.77871997289447,8.25000000000002,-1.77871997289447));
#7943=CARTESIAN_POINT('Ctrl Pts',(1.77871997289447,8.24999999999999,-4.85722573273578E-16));
#7944=CARTESIAN_POINT('Ctrl Pts',(1.77871997289447,8.24999999999997,1.77871997289447));
#7945=CARTESIAN_POINT('Ctrl Pts',(1.46367293285559E-17,8.24999999999998,
1.77871997289447));
#7946=CARTESIAN_POINT('Ctrl Pts',(-1.40833769209538E-15,7.74999999999995,
1.59062243825054));
#7947=CARTESIAN_POINT('Ctrl Pts',(-1.59062243825055,7.74999999999996,1.59062243825054));
#7948=CARTESIAN_POINT('Ctrl Pts',(-1.59062243825055,7.74999999999998,-7.62384977183021E-15));
#7949=CARTESIAN_POINT('Ctrl Pts',(-1.59062243825055,7.75,-1.59062243825056));
#7950=CARTESIAN_POINT('Ctrl Pts',(-1.40833769209538E-15,7.75,-1.59062243825056));
#7951=CARTESIAN_POINT('Ctrl Pts',(1.59062243825055,7.74999999999999,-1.59062243825056));
#7952=CARTESIAN_POINT('Ctrl Pts',(1.59062243825055,7.74999999999997,-7.62384977183034E-15));
#7953=CARTESIAN_POINT('Ctrl Pts',(1.59062243825055,7.74999999999995,1.59062243825054));
#7954=CARTESIAN_POINT('Ctrl Pts',(-1.40833769209538E-15,7.74999999999995,
1.59062243825054));
#7955=CARTESIAN_POINT('',(-1.9479506776555E-16,7.75,1.59062243825056));
#7956=CARTESIAN_POINT('Origin',(0.,7.75,0.));
#7957=CARTESIAN_POINT('',(-1.9479506776555E-16,8.75,1.59062243825056));
#7958=CARTESIAN_POINT('Origin',(-1.7390814467874E-17,8.25,0.261524741817209));
#7959=CARTESIAN_POINT('Origin',(0.,8.75,0.));
#7960=CARTESIAN_POINT('Origin',(0.,8.25,-5.52943107967607E-15));
#7961=CARTESIAN_POINT('',(-1.49484711634152,8.25,-5.34636510605184E-15));
#7962=CARTESIAN_POINT('',(1.49484711634152,8.25,-5.52943107967607E-15));
#7963=CARTESIAN_POINT('Origin',(0.,8.25,-5.52943107967607E-15));
#7964=CARTESIAN_POINT('',(0.,7.75,-1.40874692590067));
#7965=CARTESIAN_POINT('Origin',(0.,7.75,0.));
#7966=CARTESIAN_POINT('',(0.,8.75,-1.40874692590067));
#7967=CARTESIAN_POINT('Origin',(0.,8.75,0.));
#7968=CARTESIAN_POINT('Origin',(0.,8.75,-1.40874692590067));
#7969=CARTESIAN_POINT('Origin',(0.,7.75,-1.59062243825056));
#7970=CARTESIAN_POINT('Ctrl Pts',(4.37500000000006,7.57772228311413,1.59062243825047));
#7971=CARTESIAN_POINT('Ctrl Pts',(2.99748056064553,8.37303350223928,1.5906224382504));
#7972=CARTESIAN_POINT('Ctrl Pts',(2.99748056064553,8.37303350223915,-9.98890215194051E-14));
#7973=CARTESIAN_POINT('Ctrl Pts',(2.99748056064553,8.37303350223902,-1.5906224382506));
#7974=CARTESIAN_POINT('Ctrl Pts',(4.37500000000006,7.57772228311387,-1.59062243825054));
#7975=CARTESIAN_POINT('Ctrl Pts',(5.7525194393546,6.78241106398871,-1.59062243825047));
#7976=CARTESIAN_POINT('Ctrl Pts',(5.7525194393546,6.78241106398884,2.79353679939059E-14));
#7977=CARTESIAN_POINT('Ctrl Pts',(5.7525194393546,6.78241106398897,1.59062243825053));
#7978=CARTESIAN_POINT('Ctrl Pts',(4.37500000000006,7.57772228311413,1.59062243825047));
#7979=CARTESIAN_POINT('Ctrl Pts',(4.12500000000001,7.14470958122175,1.77871997289453));
#7980=CARTESIAN_POINT('Ctrl Pts',(2.58458331725451,8.03406956766891,1.77871997289446));
#7981=CARTESIAN_POINT('Ctrl Pts',(2.58458331725451,8.03406956766877,-7.20914159458848E-14));
#7982=CARTESIAN_POINT('Ctrl Pts',(2.58458331725451,8.03406956766863,-1.7787199728946));
#7983=CARTESIAN_POINT('Ctrl Pts',(4.12500000000001,7.14470958122147,-1.77871997289453));
#7984=CARTESIAN_POINT('Ctrl Pts',(5.6654166827455,6.25534959477431,-1.77871997289446));
#7985=CARTESIAN_POINT('Ctrl Pts',(5.6654166827455,6.25534959477445,7.01658728875515E-14));
#7986=CARTESIAN_POINT('Ctrl Pts',(5.6654166827455,6.25534959477459,1.7787199728946));
#7987=CARTESIAN_POINT('Ctrl Pts',(4.12500000000001,7.14470958122175,1.77871997289453));
#7988=CARTESIAN_POINT('Ctrl Pts',(3.87499999999995,6.71169687932936,1.59062243825053));
#7989=CARTESIAN_POINT('Ctrl Pts',(2.49748056064542,7.50700809845451,1.59062243825047));
#7990=CARTESIAN_POINT('Ctrl Pts',(2.49748056064542,7.50700809845438,-2.98609110522392E-14));
#7991=CARTESIAN_POINT('Ctrl Pts',(2.49748056064542,7.50700809845425,-1.59062243825053));
#7992=CARTESIAN_POINT('Ctrl Pts',(3.87499999999995,6.7116968793291,-1.59062243825046));
#7993=CARTESIAN_POINT('Ctrl Pts',(5.25251943935448,5.91638566020395,-1.5906224382504));
#7994=CARTESIAN_POINT('Ctrl Pts',(5.25251943935448,5.91638566020407,9.79634784610718E-14));
#7995=CARTESIAN_POINT('Ctrl Pts',(5.25251943935448,5.9163856602042,1.59062243825059));
#7996=CARTESIAN_POINT('Ctrl Pts',(3.87499999999995,6.71169687932936,1.59062243825053));
#7997=CARTESIAN_POINT('',(3.87500000000001,6.71169687932939,1.59062243825056));
#7998=CARTESIAN_POINT('Origin',(3.87500000000001,6.71169687932939,1.90733188991095E-16));
#7999=CARTESIAN_POINT('',(4.37500000000001,7.57772228311383,1.59062243825056));
#8000=CARTESIAN_POINT('Origin',(4.12500000000001,7.14470958122164,0.261524741817169));
#8001=CARTESIAN_POINT('Origin',(4.37500000000001,7.57772228311383,2.15343923054462E-16));
#8002=CARTESIAN_POINT('Origin',(4.12500000000001,7.14470958122162,-5.32639252365329E-15));
#8003=CARTESIAN_POINT('',(2.83042442247434,7.89213313939238,-5.23485953684118E-15));
#8004=CARTESIAN_POINT('',(5.41957557752568,6.39728602305086,-5.23485953684118E-15));
#8005=CARTESIAN_POINT('Origin',(4.12500000000001,7.14470958122162,-5.32639252365329E-15));
#8006=CARTESIAN_POINT('',(3.87500000000001,6.71169687932939,-1.40874692590067));
#8007=CARTESIAN_POINT('Origin',(3.87500000000001,6.71169687932939,1.90733188991095E-16));
#8008=CARTESIAN_POINT('',(4.37500000000001,7.57772228311383,-1.40874692590067));
#8009=CARTESIAN_POINT('Origin',(4.37500000000001,7.57772228311383,2.15343923054462E-16));
#8010=CARTESIAN_POINT('Origin',(4.37500000000001,7.57772228311383,-1.40874692590067));
#8011=CARTESIAN_POINT('Origin',(3.87500000000001,6.71169687932939,-1.59062243825056));
#8012=CARTESIAN_POINT('Ctrl Pts',(7.57772228311385,4.37500000000001,-1.59062243825054));
#8013=CARTESIAN_POINT('Ctrl Pts',(8.37303350223914,2.99748056064552,-1.59062243825056));
#8014=CARTESIAN_POINT('Ctrl Pts',(8.37303350223917,2.99748056064552,-2.03075013256419E-14));
#8015=CARTESIAN_POINT('Ctrl Pts',(8.3730335022392,2.99748056064552,1.59062243825052));
#8016=CARTESIAN_POINT('Ctrl Pts',(7.57772228311391,4.37500000000001,1.59062243825053));
#8017=CARTESIAN_POINT('Ctrl Pts',(6.78241106398862,5.75251943935451,1.59062243825055));
#8018=CARTESIAN_POINT('Ctrl Pts',(6.78241106398859,5.75251943935451,1.063000168243E-14));
#8019=CARTESIAN_POINT('Ctrl Pts',(6.78241106398856,5.75251943935451,-1.59062243825053));
#8020=CARTESIAN_POINT('Ctrl Pts',(7.57772228311385,4.37500000000001,-1.59062243825054));
#8021=CARTESIAN_POINT('Ctrl Pts',(7.1447095812216,4.12499999999999,-1.77871997289447));
#8022=CARTESIAN_POINT('Ctrl Pts',(8.03406956766886,2.58458331725462,-1.77871997289449));
#8023=CARTESIAN_POINT('Ctrl Pts',(8.03406956766889,2.58458331725462,-1.42717923056121E-14));
#8024=CARTESIAN_POINT('Ctrl Pts',(8.03406956766893,2.58458331725462,1.77871997289446));
#8025=CARTESIAN_POINT('Ctrl Pts',(7.14470958122166,4.12499999999999,1.77871997289448));
#8026=CARTESIAN_POINT('Ctrl Pts',(6.2553495947744,5.66541668274535,1.7787199728945));
#8027=CARTESIAN_POINT('Ctrl Pts',(6.25534959477437,5.66541668274535,2.11066028009605E-14));
#8028=CARTESIAN_POINT('Ctrl Pts',(6.25534959477433,5.66541668274535,-1.77871997289445));
#8029=CARTESIAN_POINT('Ctrl Pts',(7.1447095812216,4.12499999999999,-1.77871997289447));
#8030=CARTESIAN_POINT('Ctrl Pts',(6.71169687932935,3.87499999999996,-1.59062243825053));
#8031=CARTESIAN_POINT('Ctrl Pts',(7.50700809845464,2.49748056064546,-1.59062243825054));
#8032=CARTESIAN_POINT('Ctrl Pts',(7.50700809845467,2.49748056064546,-4.35030269939418E-15));
#8033=CARTESIAN_POINT('Ctrl Pts',(7.5070080984547,2.49748056064546,1.59062243825054));
#8034=CARTESIAN_POINT('Ctrl Pts',(6.71169687932941,3.87499999999996,1.59062243825055));
#8035=CARTESIAN_POINT('Ctrl Pts',(5.91638566020411,5.25251943935446,1.59062243825057));
#8036=CARTESIAN_POINT('Ctrl Pts',(5.91638566020408,5.25251943935446,2.76974233333029E-14));
#8037=CARTESIAN_POINT('Ctrl Pts',(5.91638566020405,5.25251943935446,-1.59062243825051));
#8038=CARTESIAN_POINT('Ctrl Pts',(6.71169687932935,3.87499999999996,-1.59062243825053));
#8039=CARTESIAN_POINT('',(6.7116968793294,3.87499999999999,-1.59062243825056));
#8040=CARTESIAN_POINT('Origin',(6.71169687932941,3.87499999999998,7.11825952004402E-16));
#8041=CARTESIAN_POINT('',(7.57772228311384,4.37500000000001,-1.59062243825056));
#8042=CARTESIAN_POINT('Origin',(7.14470958122162,4.12499999999998,-0.261524741817215));
#8043=CARTESIAN_POINT('Origin',(7.57772228311385,4.37499999999998,8.03674461940454E-16));
#8044=CARTESIAN_POINT('Origin',(7.14470958122163,4.12499999999998,-4.77168087270365E-15));
#8045=CARTESIAN_POINT('',(6.39728602305087,5.41957557752565,-4.68014788589154E-15));
#8046=CARTESIAN_POINT('',(7.89213313939239,2.83042442247431,-4.68014788589154E-15));
#8047=CARTESIAN_POINT('Origin',(7.14470958122163,4.12499999999998,-4.77168087270365E-15));
#8048=CARTESIAN_POINT('',(6.71169687932941,3.87499999999998,-1.40874692590067));
#8049=CARTESIAN_POINT('Origin',(6.71169687932941,3.87499999999998,7.11825952004402E-16));
#8050=CARTESIAN_POINT('',(7.57772228311385,4.37499999999998,-1.40874692590067));
#8051=CARTESIAN_POINT('Origin',(7.57772228311385,4.37499999999998,8.03674461940454E-16));
#8052=CARTESIAN_POINT('Origin',(7.57772228311385,4.37499999999998,-1.40874692590067));
#8053=CARTESIAN_POINT('Origin',(6.71169687932941,3.87499999999998,-1.59062243825056));
#8054=CARTESIAN_POINT('Ctrl Pts',(8.7500000000001,-3.01501838019841E-14,
-1.59062243825053));
#8055=CARTESIAN_POINT('Ctrl Pts',(8.75000000000009,-1.59062243825058,-1.59062243825053));
#8056=CARTESIAN_POINT('Ctrl Pts',(8.75000000000004,-1.59062243825058,1.7123474122469E-14));
#8057=CARTESIAN_POINT('Ctrl Pts',(8.75,-1.59062243825058,1.59062243825056));
#8058=CARTESIAN_POINT('Ctrl Pts',(8.75,-3.01501838019841E-14,1.59062243825056));
#8059=CARTESIAN_POINT('Ctrl Pts',(8.75000000000001,1.59062243825052,1.59062243825056));
#8060=CARTESIAN_POINT('Ctrl Pts',(8.75000000000006,1.59062243825052,1.71234741224694E-14));
#8061=CARTESIAN_POINT('Ctrl Pts',(8.7500000000001,1.59062243825052,-1.59062243825053));
#8062=CARTESIAN_POINT('Ctrl Pts',(8.7500000000001,-3.01501838019841E-14,
-1.59062243825053));
#8063=CARTESIAN_POINT('Ctrl Pts',(8.25000000000005,-2.83665235398244E-14,
-1.77871997289448));
#8064=CARTESIAN_POINT('Ctrl Pts',(8.25000000000005,-1.77871997289451,-1.77871997289448));
#8065=CARTESIAN_POINT('Ctrl Pts',(8.24999999999999,-1.77871997289451,2.08166817117158E-15));
#8066=CARTESIAN_POINT('Ctrl Pts',(8.24999999999994,-1.77871997289451,1.77871997289448));
#8067=CARTESIAN_POINT('Ctrl Pts',(8.24999999999995,-2.83665235398245E-14,
1.77871997289448));
#8068=CARTESIAN_POINT('Ctrl Pts',(8.24999999999995,1.77871997289445,1.77871997289448));
#8069=CARTESIAN_POINT('Ctrl Pts',(8.25000000000001,1.77871997289445,2.08166817117197E-15));
#8070=CARTESIAN_POINT('Ctrl Pts',(8.25000000000006,1.77871997289445,-1.77871997289448));
#8071=CARTESIAN_POINT('Ctrl Pts',(8.25000000000005,-2.83665235398244E-14,
-1.77871997289448));
#8072=CARTESIAN_POINT('Ctrl Pts',(7.75,-2.65828632776648E-14,-1.59062243825055));
#8073=CARTESIAN_POINT('Ctrl Pts',(7.75,-1.59062243825056,-1.59062243825055));
#8074=CARTESIAN_POINT('Ctrl Pts',(7.74999999999995,-1.59062243825056,-1.29601377801257E-14));
#8075=CARTESIAN_POINT('Ctrl Pts',(7.7499999999999,-1.59062243825056,1.59062243825052));
#8076=CARTESIAN_POINT('Ctrl Pts',(7.74999999999991,-2.65828632776648E-14,
1.59062243825052));
#8077=CARTESIAN_POINT('Ctrl Pts',(7.74999999999991,1.59062243825051,1.59062243825052));
#8078=CARTESIAN_POINT('Ctrl Pts',(7.74999999999996,1.59062243825051,-1.29601377801253E-14));
#8079=CARTESIAN_POINT('Ctrl Pts',(7.75000000000001,1.59062243825051,-1.59062243825055));
#8080=CARTESIAN_POINT('Ctrl Pts',(7.75,-2.65828632776648E-14,-1.59062243825055));
#8081=CARTESIAN_POINT('',(7.75,-2.67776583454304E-14,-1.59062243825056));
#8082=CARTESIAN_POINT('Origin',(7.75,-2.70589803760343E-14,1.4236519040088E-15));
#8083=CARTESIAN_POINT('',(8.75,-3.03449788697493E-14,-1.59062243825056));
#8084=CARTESIAN_POINT('Origin',(8.25000000000002,-2.83985510836209E-14,
-0.261524741817196));
#8085=CARTESIAN_POINT('Origin',(8.75,-3.05504617148774E-14,1.60734892388091E-15));
#8086=CARTESIAN_POINT('Origin',(8.25,-2.88047210454559E-14,-4.01393066573122E-15));
#8087=CARTESIAN_POINT('',(8.25000000000001,1.49484711634149,-4.10546365254334E-15));
#8088=CARTESIAN_POINT('',(8.24999999999999,-1.49484711634155,-3.73933170529488E-15));
#8089=CARTESIAN_POINT('Origin',(8.25,-2.88047210454559E-14,-4.01393066573122E-15));
#8090=CARTESIAN_POINT('',(7.75,-2.73177629880762E-14,-1.40874692590067));
#8091=CARTESIAN_POINT('Origin',(7.75,-2.70589803760343E-14,1.4236519040088E-15));
#8092=CARTESIAN_POINT('',(8.75,-3.08092443269194E-14,-1.40874692590067));
#8093=CARTESIAN_POINT('Origin',(8.75,-3.05504617148774E-14,1.60734892388091E-15));
#8094=CARTESIAN_POINT('Origin',(8.75,-3.08092443269194E-14,-1.40874692590067));
#8095=CARTESIAN_POINT('Origin',(7.75,-2.73511729776826E-14,-1.59062243825056));
#8096=CARTESIAN_POINT('Ctrl Pts',(7.57772228311398,-4.37500000000007,-1.5906224382505));
#8097=CARTESIAN_POINT('Ctrl Pts',(6.78241106398874,-5.75251943935458,-1.59062243825054));
#8098=CARTESIAN_POINT('Ctrl Pts',(6.78241106398865,-5.75251943935458,-1.83119572337645E-14));
#8099=CARTESIAN_POINT('Ctrl Pts',(6.78241106398857,-5.75251943935458,1.59062243825051));
#8100=CARTESIAN_POINT('Ctrl Pts',(7.57772228311382,-4.37500000000007,1.59062243825055));
#8101=CARTESIAN_POINT('Ctrl Pts',(8.37303350223906,-2.99748056064556,1.59062243825059));
#8102=CARTESIAN_POINT('Ctrl Pts',(8.37303350223915,-2.99748056064556,6.49547696131205E-14));
#8103=CARTESIAN_POINT('Ctrl Pts',(8.37303350223923,-2.99748056064556,-1.59062243825046));
#8104=CARTESIAN_POINT('Ctrl Pts',(7.57772228311398,-4.37500000000007,-1.5906224382505));
#8105=CARTESIAN_POINT('Ctrl Pts',(7.1447095812217,-4.12500000000003,-1.7787199728945));
#8106=CARTESIAN_POINT('Ctrl Pts',(6.25534959477447,-5.66541668274545,-1.77871997289454));
#8107=CARTESIAN_POINT('Ctrl Pts',(6.25534959477437,-5.66541668274545,-4.55067786765486E-14));
#8108=CARTESIAN_POINT('Ctrl Pts',(6.25534959477428,-5.66541668274545,1.77871997289445));
#8109=CARTESIAN_POINT('Ctrl Pts',(7.14470958122151,-4.12500000000003,1.7787199728945));
#8110=CARTESIAN_POINT('Ctrl Pts',(8.03406956766874,-2.58458331725462,1.77871997289454));
#8111=CARTESIAN_POINT('Ctrl Pts',(8.03406956766883,-2.58458331725462,4.67904740487708E-14));
#8112=CARTESIAN_POINT('Ctrl Pts',(8.03406956766892,-2.58458331725462,-1.77871997289445));
#8113=CARTESIAN_POINT('Ctrl Pts',(7.1447095812217,-4.12500000000003,-1.7787199728945));
#8114=CARTESIAN_POINT('Ctrl Pts',(6.71169687932939,-3.875,-1.59062243825054));
#8115=CARTESIAN_POINT('Ctrl Pts',(5.91638566020415,-5.2525194393545,-1.59062243825058));
#8116=CARTESIAN_POINT('Ctrl Pts',(5.91638566020406,-5.2525194393545,-6.31903335693023E-14));
#8117=CARTESIAN_POINT('Ctrl Pts',(5.91638566020398,-5.2525194393545,1.59062243825046));
#8118=CARTESIAN_POINT('Ctrl Pts',(6.71169687932922,-3.875,1.5906224382505));
#8119=CARTESIAN_POINT('Ctrl Pts',(7.50700809845447,-2.49748056064549,1.59062243825054));
#8120=CARTESIAN_POINT('Ctrl Pts',(7.50700809845455,-2.49748056064549,1.91149119343909E-14));
#8121=CARTESIAN_POINT('Ctrl Pts',(7.50700809845463,-2.49748056064549,-1.5906224382505));
#8122=CARTESIAN_POINT('Ctrl Pts',(6.71169687932939,-3.875,-1.59062243825054));
#8123=CARTESIAN_POINT('',(6.7116968793294,-3.875,-1.59062243825056));
#8124=CARTESIAN_POINT('Origin',(6.71169687932938,-3.87500000000003,2.1354778560132E-15));
#8125=CARTESIAN_POINT('',(7.57772228311385,-4.37499999999999,-1.59062243825056));
#8126=CARTESIAN_POINT('Origin',(7.14470958122162,-4.12500000000004,-0.261524741817231));
#8127=CARTESIAN_POINT('Origin',(7.57772228311382,-4.37500000000004,2.41102338582136E-15));
#8128=CARTESIAN_POINT('Origin',(7.1447095812216,-4.12500000000003,-3.25618045875879E-15));
#8129=CARTESIAN_POINT('',(7.89213313939237,-2.83042442247437,-3.16464747194668E-15));
#8130=CARTESIAN_POINT('',(6.39728602305083,-5.41957557752569,-3.16464747194668E-15));
#8131=CARTESIAN_POINT('Origin',(7.1447095812216,-4.12500000000003,-3.25618045875879E-15));
#8132=CARTESIAN_POINT('',(6.71169687932938,-3.87500000000003,-1.40874692590067));
#8133=CARTESIAN_POINT('Origin',(6.71169687932938,-3.87500000000003,2.1354778560132E-15));
#8134=CARTESIAN_POINT('',(7.57772228311382,-4.37500000000004,-1.40874692590067));
#8135=CARTESIAN_POINT('Origin',(7.57772228311382,-4.37500000000004,2.41102338582136E-15));
#8136=CARTESIAN_POINT('Origin',(7.57772228311382,-4.37500000000004,-1.40874692590067));
#8137=CARTESIAN_POINT('Origin',(6.71169687932938,-3.87500000000003,-1.59062243825055));
#8138=CARTESIAN_POINT('Ctrl Pts',(4.37499999999984,-7.57772228311397,-1.59062243825053));
#8139=CARTESIAN_POINT('Ctrl Pts',(2.99748056064537,-8.37303350223927,-1.59062243825036));
#8140=CARTESIAN_POINT('Ctrl Pts',(2.99748056064557,-8.37303350223927,1.48340183158392E-13));
#8141=CARTESIAN_POINT('Ctrl Pts',(2.99748056064577,-8.37303350223927,1.59062243825066));
#8142=CARTESIAN_POINT('Ctrl Pts',(4.37500000000023,-7.57772228311397,1.59062243825049));
#8143=CARTESIAN_POINT('Ctrl Pts',(5.7525194393547,-6.78241106398868,1.59062243825031));
#8144=CARTESIAN_POINT('Ctrl Pts',(5.7525194393545,-6.78241106398868,-1.96831619047452E-13));
#8145=CARTESIAN_POINT('Ctrl Pts',(5.7525194393543,-6.78241106398868,-1.59062243825071));
#8146=CARTESIAN_POINT('Ctrl Pts',(4.37499999999984,-7.57772228311397,-1.59062243825053));
#8147=CARTESIAN_POINT('Ctrl Pts',(4.12499999999973,-7.14470958122165,-1.7787199728945));
#8148=CARTESIAN_POINT('Ctrl Pts',(2.58458331725435,-8.03406956766895,-1.77871997289431));
#8149=CARTESIAN_POINT('Ctrl Pts',(2.58458331725457,-8.03406956766895,1.99898049178834E-13));
#8150=CARTESIAN_POINT('Ctrl Pts',(2.58458331725479,-8.03406956766895,1.77871997289471));
#8151=CARTESIAN_POINT('Ctrl Pts',(4.12500000000018,-7.14470958122165,1.77871997289452));
#8152=CARTESIAN_POINT('Ctrl Pts',(5.66541668274557,-6.25534959477435,1.77871997289432));
#8153=CARTESIAN_POINT('Ctrl Pts',(5.66541668274534,-6.25534959477435,-1.85655969441064E-13));
#8154=CARTESIAN_POINT('Ctrl Pts',(5.66541668274512,-6.25534959477435,-1.7787199728947));
#8155=CARTESIAN_POINT('Ctrl Pts',(4.12499999999973,-7.14470958122165,-1.7787199728945));
#8156=CARTESIAN_POINT('Ctrl Pts',(3.87499999999968,-6.71169687932932,-1.59062243825047));
#8157=CARTESIAN_POINT('Ctrl Pts',(2.49748056064522,-7.50700809845462,-1.5906224382503));
#8158=CARTESIAN_POINT('Ctrl Pts',(2.49748056064542,-7.50700809845462,2.11073698785222E-13));
#8159=CARTESIAN_POINT('Ctrl Pts',(2.49748056064561,-7.50700809845462,1.59062243825072));
#8160=CARTESIAN_POINT('Ctrl Pts',(3.87500000000008,-6.71169687932932,1.59062243825055));
#8161=CARTESIAN_POINT('Ctrl Pts',(5.25251943935454,-5.91638566020402,1.59062243825038));
#8162=CARTESIAN_POINT('Ctrl Pts',(5.25251943935434,-5.91638566020402,-1.34098103420622E-13));
#8163=CARTESIAN_POINT('Ctrl Pts',(5.25251943935414,-5.91638566020402,-1.59062243825064));
#8164=CARTESIAN_POINT('Ctrl Pts',(3.87499999999968,-6.71169687932932,-1.59062243825047));
#8165=CARTESIAN_POINT('',(3.87499999999979,-6.71169687932952,-1.59062243825056));
#8166=CARTESIAN_POINT('Origin',(3.87499999999996,-6.71169687932942,2.65657061902651E-15));
#8167=CARTESIAN_POINT('',(4.37499999999982,-7.57772228311395,-1.59062243825056));
#8168=CARTESIAN_POINT('Origin',(4.12499999999992,-7.14470958122165,-0.261524741817159));
#8169=CARTESIAN_POINT('Origin',(4.37499999999996,-7.57772228311387,2.99935392470735E-15));
#8170=CARTESIAN_POINT('Origin',(4.12499999999996,-7.14470958122164,-2.70146880780915E-15));
#8171=CARTESIAN_POINT('',(5.41957557752563,-6.39728602305089,-3.16504733330961E-15));
#8172=CARTESIAN_POINT('',(2.83042442247429,-7.89213313939239,-2.05482430868446E-15));
#8173=CARTESIAN_POINT('Origin',(4.12499999999996,-7.14470958122164,-2.70146880780915E-15));
#8174=CARTESIAN_POINT('',(3.87499999999996,-6.71169687932942,-1.40874692590067));
#8175=CARTESIAN_POINT('Origin',(3.87499999999996,-6.71169687932942,2.65657061902651E-15));
#8176=CARTESIAN_POINT('',(4.37499999999996,-7.57772228311387,-1.40874692590067));
#8177=CARTESIAN_POINT('Origin',(4.37499999999996,-7.57772228311387,2.99935392470735E-15));
#8178=CARTESIAN_POINT('Origin',(4.37499999999996,-7.57772228311387,-1.40874692590067));
#8179=CARTESIAN_POINT('Origin',(3.87499999999996,-6.71169687932942,-1.59062243825055));
#8180=CARTESIAN_POINT('Ctrl Pts',(3.82926740629614E-15,-8.75000000000001,
-1.59062243825056));
#8181=CARTESIAN_POINT('Ctrl Pts',(-1.59062243825054,-8.75000000000002,-1.59062243825056));
#8182=CARTESIAN_POINT('Ctrl Pts',(-1.59062243825054,-8.75000000000005,-9.87978730961784E-15));
#8183=CARTESIAN_POINT('Ctrl Pts',(-1.59062243825054,-8.75000000000008,1.59062243825054));
#8184=CARTESIAN_POINT('Ctrl Pts',(3.82926740629613E-15,-8.75000000000007,
1.59062243825054));
#8185=CARTESIAN_POINT('Ctrl Pts',(1.59062243825055,-8.75000000000006,1.59062243825054));
#8186=CARTESIAN_POINT('Ctrl Pts',(1.59062243825055,-8.75000000000003,-9.87978730961739E-15));
#8187=CARTESIAN_POINT('Ctrl Pts',(1.59062243825055,-8.75,-1.59062243825056));
#8188=CARTESIAN_POINT('Ctrl Pts',(3.82926740629614E-15,-8.75000000000001,
-1.59062243825056));
#8189=CARTESIAN_POINT('Ctrl Pts',(1.01372903127415E-16,-8.24999999999997,
-1.77871997289448));
#8190=CARTESIAN_POINT('Ctrl Pts',(-1.77871997289448,-8.24999999999998,-1.77871997289448));
#8191=CARTESIAN_POINT('Ctrl Pts',(-1.77871997289448,-8.25000000000001,-3.20923843056017E-16));
#8192=CARTESIAN_POINT('Ctrl Pts',(-1.77871997289448,-8.25000000000005,1.77871997289448));
#8193=CARTESIAN_POINT('Ctrl Pts',(1.01372903127413E-16,-8.25000000000004,
1.77871997289448));
#8194=CARTESIAN_POINT('Ctrl Pts',(1.77871997289448,-8.25000000000002,1.77871997289448));
#8195=CARTESIAN_POINT('Ctrl Pts',(1.77871997289448,-8.24999999999999,-3.20923843055502E-16));
#8196=CARTESIAN_POINT('Ctrl Pts',(1.77871997289448,-8.24999999999995,-1.77871997289448));
#8197=CARTESIAN_POINT('Ctrl Pts',(1.01372903127415E-16,-8.24999999999997,
-1.77871997289448));
#8198=CARTESIAN_POINT('Ctrl Pts',(-3.6265216000413E-15,-7.74999999999993,
-1.59062243825054));
#8199=CARTESIAN_POINT('Ctrl Pts',(-1.59062243825055,-7.74999999999995,-1.59062243825054));
#8200=CARTESIAN_POINT('Ctrl Pts',(-1.59062243825055,-7.74999999999998,9.23793962350586E-15));
#8201=CARTESIAN_POINT('Ctrl Pts',(-1.59062243825055,-7.75000000000001,1.59062243825056));
#8202=CARTESIAN_POINT('Ctrl Pts',(-3.62652160004131E-15,-7.74999999999999,
1.59062243825056));
#8203=CARTESIAN_POINT('Ctrl Pts',(1.59062243825055,-7.74999999999998,1.59062243825056));
#8204=CARTESIAN_POINT('Ctrl Pts',(1.59062243825055,-7.74999999999995,9.23793962350631E-15));
#8205=CARTESIAN_POINT('Ctrl Pts',(1.59062243825055,-7.74999999999992,-1.59062243825054));
#8206=CARTESIAN_POINT('Ctrl Pts',(-3.6265216000413E-15,-7.74999999999993,
-1.59062243825054));
#8207=CARTESIAN_POINT('',(-3.82131666780635E-15,-7.75,-1.59062243825056));
#8208=CARTESIAN_POINT('Origin',(0.,-7.75,2.8473038080176E-15));
#8209=CARTESIAN_POINT('',(3.63447233853054E-15,-8.75,-1.59062243825056));
#8210=CARTESIAN_POINT('Origin',(6.9345359330968E-17,-8.24999999999999,-0.261524741817196));
#8211=CARTESIAN_POINT('Origin',(0.,-8.75,3.2146978477618E-15));
#8212=CARTESIAN_POINT('Origin',(0.,-8.25,-2.49843025178637E-15));
#8213=CARTESIAN_POINT('',(1.49484711634152,-8.25,-2.31536427816214E-15));
#8214=CARTESIAN_POINT('',(-1.49484711634152,-8.25,-2.49843025178637E-15));
#8215=CARTESIAN_POINT('Origin',(0.,-8.25,-2.49843025178637E-15));
#8216=CARTESIAN_POINT('',(0.,-7.75,-1.40874692590067));
#8217=CARTESIAN_POINT('Origin',(0.,-7.75,2.8473038080176E-15));
#8218=CARTESIAN_POINT('',(0.,-8.75,-1.40874692590067));
#8219=CARTESIAN_POINT('Origin',(0.,-8.75,3.2146978477618E-15));
#8220=CARTESIAN_POINT('Origin',(0.,-8.75,-1.40874692590067));
#8221=CARTESIAN_POINT('Origin',(0.,-7.75,-1.59062243825055));
#8222=CARTESIAN_POINT('Ctrl Pts',(-4.37500000000018,-7.57772228311385,1.59062243825053));
#8223=CARTESIAN_POINT('Ctrl Pts',(-2.9974805606457,-8.37303350223915,1.5906224382506));
#8224=CARTESIAN_POINT('Ctrl Pts',(-2.99748056064561,-8.37303350223915,6.28013398870636E-14));
#8225=CARTESIAN_POINT('Ctrl Pts',(-2.99748056064553,-8.37303350223915,-1.59062243825047));
#8226=CARTESIAN_POINT('Ctrl Pts',(-4.37500000000001,-7.57772228311385,-1.59062243825055));
#8227=CARTESIAN_POINT('Ctrl Pts',(-5.7525194393545,-6.78241106398854,-1.59062243825062));
#8228=CARTESIAN_POINT('Ctrl Pts',(-5.75251943935459,-6.78241106398854,-8.52667869644686E-14));
#8229=CARTESIAN_POINT('Ctrl Pts',(-5.75251943935467,-6.78241106398854,1.59062243825045));
#8230=CARTESIAN_POINT('Ctrl Pts',(-4.37500000000018,-7.57772228311385,1.59062243825053));
#8231=CARTESIAN_POINT('Ctrl Pts',(-4.12500000000016,-7.14470958122159,1.77871997289448));
#8232=CARTESIAN_POINT('Ctrl Pts',(-2.58458331725479,-8.03406956766887,1.77871997289457));
#8233=CARTESIAN_POINT('Ctrl Pts',(-2.58458331725469,-8.03406956766887,8.49165151811221E-14));
#8234=CARTESIAN_POINT('Ctrl Pts',(-2.5845833172546,-8.03406956766887,-1.7787199728944));
#8235=CARTESIAN_POINT('Ctrl Pts',(-4.12499999999996,-7.14470958122159,-1.77871997289448));
#8236=CARTESIAN_POINT('Ctrl Pts',(-5.66541668274533,-6.2553495947743,-1.77871997289456));
#8237=CARTESIAN_POINT('Ctrl Pts',(-5.66541668274543,-6.2553495947743,-8.04582758478618E-14));
#8238=CARTESIAN_POINT('Ctrl Pts',(-5.66541668274552,-6.2553495947743,1.7787199728944));
#8239=CARTESIAN_POINT('Ctrl Pts',(-4.12500000000016,-7.14470958122159,1.77871997289448));
#8240=CARTESIAN_POINT('Ctrl Pts',(-3.87500000000011,-6.71169687932933,1.59062243825055));
#8241=CARTESIAN_POINT('Ctrl Pts',(-2.49748056064562,-7.50700809845463,1.59062243825063));
#8242=CARTESIAN_POINT('Ctrl Pts',(-2.49748056064553,-7.50700809845463,8.97250262977289E-14));
#8243=CARTESIAN_POINT('Ctrl Pts',(-2.49748056064545,-7.50700809845463,-1.59062243825045));
#8244=CARTESIAN_POINT('Ctrl Pts',(-3.87499999999994,-6.71169687932933,-1.59062243825052));
#8245=CARTESIAN_POINT('Ctrl Pts',(-5.25251943935443,-5.91638566020402,-1.5906224382506));
#8246=CARTESIAN_POINT('Ctrl Pts',(-5.25251943935451,-5.91638566020402,-5.83431005538033E-14));
#8247=CARTESIAN_POINT('Ctrl Pts',(-5.2525194393546,-5.91638566020402,1.59062243825048));
#8248=CARTESIAN_POINT('Ctrl Pts',(-3.87500000000011,-6.71169687932933,1.59062243825055));
#8249=CARTESIAN_POINT('',(-3.87500000000006,-6.71169687932937,1.59062243825056));
#8250=CARTESIAN_POINT('Origin',(-3.87500000000006,-6.71169687932937,2.6565706190265E-15));
#8251=CARTESIAN_POINT('',(-4.37500000000006,-7.5777222831138,1.59062243825056));
#8252=CARTESIAN_POINT('Origin',(-4.12500000000007,-7.14470958122158,0.261524741817216));
#8253=CARTESIAN_POINT('Origin',(-4.37500000000006,-7.5777222831138,2.99935392470734E-15));
#8254=CARTESIAN_POINT('Origin',(-4.12500000000006,-7.14470958122159,-2.70146880780916E-15));
#8255=CARTESIAN_POINT('',(-2.8304244224744,-7.89213313939236,-2.05482430868446E-15));
#8256=CARTESIAN_POINT('',(-5.41957557752572,-6.39728602305082,-3.16504733330963E-15));
#8257=CARTESIAN_POINT('Origin',(-4.12500000000006,-7.14470958122159,-2.70146880780916E-15));
#8258=CARTESIAN_POINT('',(-3.87500000000006,-6.71169687932937,-1.40874692590067));
#8259=CARTESIAN_POINT('Origin',(-3.87500000000006,-6.71169687932937,2.6565706190265E-15));
#8260=CARTESIAN_POINT('',(-4.37500000000006,-7.5777222831138,-1.40874692590067));
#8261=CARTESIAN_POINT('Origin',(-4.37500000000006,-7.5777222831138,2.99935392470734E-15));
#8262=CARTESIAN_POINT('Origin',(-4.37500000000006,-7.5777222831138,-1.40874692590067));
#8263=CARTESIAN_POINT('Origin',(-3.87500000000006,-6.71169687932937,-1.59062243825055));
#8264=CARTESIAN_POINT('Ctrl Pts',(-7.57772228311387,-4.37499999999996,1.59062243825055));
#8265=CARTESIAN_POINT('Ctrl Pts',(-6.78241106398862,-5.75251943935447,1.59062243825052));
#8266=CARTESIAN_POINT('Ctrl Pts',(-6.78241106398868,-5.75251943935447,-1.35911445937371E-14));
#8267=CARTESIAN_POINT('Ctrl Pts',(-6.78241106398875,-5.75251943935447,-1.59062243825055));
#8268=CARTESIAN_POINT('Ctrl Pts',(-7.577722283114,-4.37499999999996,-1.59062243825051));
#8269=CARTESIAN_POINT('Ctrl Pts',(-8.37303350223925,-2.99748056064545,-1.59062243825048));
#8270=CARTESIAN_POINT('Ctrl Pts',(-8.37303350223919,-2.99748056064545,5.28734952023379E-14));
#8271=CARTESIAN_POINT('Ctrl Pts',(-8.37303350223912,-2.99748056064545,1.59062243825059));
#8272=CARTESIAN_POINT('Ctrl Pts',(-7.57772228311387,-4.37499999999996,1.59062243825055));
#8273=CARTESIAN_POINT('Ctrl Pts',(-7.14470958122159,-4.12499999999993,1.77871997289449));
#8274=CARTESIAN_POINT('Ctrl Pts',(-6.25534959477436,-5.66541668274533,1.77871997289445));
#8275=CARTESIAN_POINT('Ctrl Pts',(-6.25534959477443,-5.66541668274533,-3.59037940510415E-14));
#8276=CARTESIAN_POINT('Ctrl Pts',(-6.25534959477451,-5.66541668274533,-1.77871997289452));
#8277=CARTESIAN_POINT('Ctrl Pts',(-7.14470958122174,-4.12499999999993,-1.77871997289448));
#8278=CARTESIAN_POINT('Ctrl Pts',(-8.03406956766896,-2.58458331725453,-1.77871997289444));
#8279=CARTESIAN_POINT('Ctrl Pts',(-8.03406956766889,-2.58458331725453,3.94426299420347E-14));
#8280=CARTESIAN_POINT('Ctrl Pts',(-8.03406956766881,-2.58458331725453,1.77871997289452));
#8281=CARTESIAN_POINT('Ctrl Pts',(-7.14470958122159,-4.12499999999993,1.77871997289449));
#8282=CARTESIAN_POINT('Ctrl Pts',(-6.71169687932932,-3.87499999999991,1.59062243825052));
#8283=CARTESIAN_POINT('Ctrl Pts',(-5.91638566020407,-5.25251943935442,1.59062243825049));
#8284=CARTESIAN_POINT('Ctrl Pts',(-5.91638566020413,-5.25251943935442,-4.93346593113448E-14));
#8285=CARTESIAN_POINT('Ctrl Pts',(-5.9163856602042,-5.25251943935442,-1.59062243825059));
#8286=CARTESIAN_POINT('Ctrl Pts',(-6.71169687932945,-3.87499999999991,-1.59062243825055));
#8287=CARTESIAN_POINT('Ctrl Pts',(-7.50700809845471,-2.49748056064539,-1.59062243825052));
#8288=CARTESIAN_POINT('Ctrl Pts',(-7.50700809845464,-2.49748056064539,1.71299804847301E-14));
#8289=CARTESIAN_POINT('Ctrl Pts',(-7.50700809845458,-2.49748056064539,1.59062243825055));
#8290=CARTESIAN_POINT('Ctrl Pts',(-6.71169687932932,-3.87499999999991,1.59062243825052));
#8291=CARTESIAN_POINT('',(-6.71169687932944,-3.87499999999994,1.59062243825056));
#8292=CARTESIAN_POINT('Origin',(-6.71169687932943,-3.87499999999994,2.13547785601319E-15));
#8293=CARTESIAN_POINT('',(-7.57772228311388,-4.37499999999993,1.59062243825056));
#8294=CARTESIAN_POINT('Origin',(-7.14470958122164,-4.12499999999993,0.261524741817217));
#8295=CARTESIAN_POINT('Origin',(-7.57772228311388,-4.37499999999993,2.41102338582134E-15));
#8296=CARTESIAN_POINT('Origin',(-7.14470958122166,-4.12499999999993,-3.25618045875881E-15));
#8297=CARTESIAN_POINT('',(-6.39728602305091,-5.41957557752561,-3.1646474719467E-15));
#8298=CARTESIAN_POINT('',(-7.89213313939241,-2.83042442247425,-3.1646474719467E-15));
#8299=CARTESIAN_POINT('Origin',(-7.14470958122166,-4.12499999999993,-3.25618045875881E-15));
#8300=CARTESIAN_POINT('',(-6.71169687932943,-3.87499999999994,-1.40874692590067));
#8301=CARTESIAN_POINT('Origin',(-6.71169687932943,-3.87499999999994,2.13547785601319E-15));
#8302=CARTESIAN_POINT('',(-7.57772228311388,-4.37499999999993,-1.40874692590067));
#8303=CARTESIAN_POINT('Origin',(-7.57772228311388,-4.37499999999993,2.41102338582134E-15));
#8304=CARTESIAN_POINT('Origin',(-7.57772228311388,-4.37499999999993,-1.40874692590067));
#8305=CARTESIAN_POINT('Origin',(-6.71169687932943,-3.87499999999994,-1.59062243825055));
#8306=CARTESIAN_POINT('Ctrl Pts',(-8.75000000000024,8.99419774478253E-14,
1.59062243825048));
#8307=CARTESIAN_POINT('Ctrl Pts',(-8.75000000000025,-1.59062243825042,1.59062243825048));
#8308=CARTESIAN_POINT('Ctrl Pts',(-8.75000000000013,-1.59062243825043,-3.5209082131642E-14));
#8309=CARTESIAN_POINT('Ctrl Pts',(-8.75000000000001,-1.59062243825042,-1.59062243825055));
#8310=CARTESIAN_POINT('Ctrl Pts',(-8.75,8.99419774478253E-14,-1.59062243825055));
#8311=CARTESIAN_POINT('Ctrl Pts',(-8.75,1.5906224382506,-1.59062243825055));
#8312=CARTESIAN_POINT('Ctrl Pts',(-8.75000000000012,1.5906224382506,-3.52090821316413E-14));
#8313=CARTESIAN_POINT('Ctrl Pts',(-8.75000000000024,1.5906224382506,1.59062243825048));
#8314=CARTESIAN_POINT('Ctrl Pts',(-8.75000000000024,8.99419774478253E-14,
1.59062243825048));
#8315=CARTESIAN_POINT('Ctrl Pts',(-8.25000000000013,8.83781979890697E-14,
1.77871997289451));
#8316=CARTESIAN_POINT('Ctrl Pts',(-8.25000000000014,-1.77871997289442,1.77871997289451));
#8317=CARTESIAN_POINT('Ctrl Pts',(-8.25000000000001,-1.77871997289442,2.65412691824407E-15));
#8318=CARTESIAN_POINT('Ctrl Pts',(-8.24999999999987,-1.77871997289442,-1.77871997289451));
#8319=CARTESIAN_POINT('Ctrl Pts',(-8.24999999999986,8.83781979890697E-14,
-1.77871997289451));
#8320=CARTESIAN_POINT('Ctrl Pts',(-8.24999999999986,1.7787199728946,-1.77871997289451));
#8321=CARTESIAN_POINT('Ctrl Pts',(-8.24999999999999,1.7787199728946,2.65412691824491E-15));
#8322=CARTESIAN_POINT('Ctrl Pts',(-8.25000000000013,1.7787199728946,1.77871997289451));
#8323=CARTESIAN_POINT('Ctrl Pts',(-8.25000000000013,8.83781979890697E-14,
1.77871997289451));
#8324=CARTESIAN_POINT('Ctrl Pts',(-7.74999999999999,8.6814418530314E-14,
1.59062243825055));
#8325=CARTESIAN_POINT('Ctrl Pts',(-7.75,-1.59062243825043,1.59062243825055));
#8326=CARTESIAN_POINT('Ctrl Pts',(-7.74999999999988,-1.59062243825043,4.05173359681304E-14));
#8327=CARTESIAN_POINT('Ctrl Pts',(-7.74999999999976,-1.59062243825043,-1.59062243825047));
#8328=CARTESIAN_POINT('Ctrl Pts',(-7.74999999999975,8.6814418530314E-14,
-1.59062243825047));
#8329=CARTESIAN_POINT('Ctrl Pts',(-7.74999999999975,1.5906224382506,-1.59062243825047));
#8330=CARTESIAN_POINT('Ctrl Pts',(-7.74999999999987,1.5906224382506,4.05173359681311E-14));
#8331=CARTESIAN_POINT('Ctrl Pts',(-7.74999999999999,1.5906224382506,1.59062243825055));
#8332=CARTESIAN_POINT('Ctrl Pts',(-7.74999999999999,8.6814418530314E-14,
1.59062243825055));
#8333=CARTESIAN_POINT('',(-7.75,8.12743386619856E-14,1.59062243825056));
#8334=CARTESIAN_POINT('Origin',(-7.75,8.11769411281028E-14,1.42365190400878E-15));
#8335=CARTESIAN_POINT('',(-8.75,9.1748782678515E-14,1.59062243825056));
#8336=CARTESIAN_POINT('Origin',(-8.25000000000002,8.83461704452732E-14,
0.261524741817187));
#8337=CARTESIAN_POINT('Origin',(-8.75,9.16513851446323E-14,1.60734892388089E-15));
#8338=CARTESIAN_POINT('Origin',(-8.25,8.64141631363676E-14,-4.01393066573124E-15));
#8339=CARTESIAN_POINT('',(-8.25000000000002,-1.49484711634143,-3.55626573167068E-15));
#8340=CARTESIAN_POINT('',(-8.24999999999999,1.49484711634161,-4.28852962616757E-15));
#8341=CARTESIAN_POINT('Origin',(-8.25,8.64141631363676E-14,-4.01393066573124E-15));
#8342=CARTESIAN_POINT('',(-7.75,8.09181585160609E-14,-1.40874692590067));
#8343=CARTESIAN_POINT('Origin',(-7.75,8.11769411281028E-14,1.42365190400878E-15));
#8344=CARTESIAN_POINT('',(-8.75,9.13926025325903E-14,-1.40874692590067));
#8345=CARTESIAN_POINT('Origin',(-8.75,9.16513851446323E-14,1.60734892388089E-15));
#8346=CARTESIAN_POINT('Origin',(-8.75,9.13926025325903E-14,-1.40874692590067));
#8347=CARTESIAN_POINT('Origin',(-7.75,8.08847485264545E-14,-1.59062243825056));
#8348=CARTESIAN_POINT('Origin',(0.,0.,-0.416666666666667));
#8349=CARTESIAN_POINT('',(8.25,-1.01033360929657E-15,0.416666666666667));
#8350=CARTESIAN_POINT('Origin',(0.,0.,0.416666666666667));
#8351=CARTESIAN_POINT('',(8.25,-1.01033360929657E-15,-0.416666666666667));
#8352=CARTESIAN_POINT('',(8.25,-1.01033360929657E-15,-0.416666666666667));
#8353=CARTESIAN_POINT('Origin',(0.,0.,-0.416666666666667));
#8354=CARTESIAN_POINT('Origin',(0.,0.,-0.416666666666667));
#8355=CARTESIAN_POINT('',(8.75,-1.07156594925393E-15,-0.416666666666667));
#8356=CARTESIAN_POINT('Origin',(0.,0.,-0.416666666666667));
#8357=CARTESIAN_POINT('',(8.75,-1.07156594925393E-15,0.416666666666667));
#8358=CARTESIAN_POINT('',(8.75,-1.07156594925393E-15,-0.416666666666667));
#8359=CARTESIAN_POINT('Origin',(0.,0.,0.416666666666667));
#8360=CARTESIAN_POINT('Origin',(0.,0.,-0.416666666666667));
#8361=CARTESIAN_POINT('Origin',(0.,0.,0.416666666666667));
#8362=CARTESIAN_POINT('Ctrl Pts',(-7.57772228311383,4.3750000000001,1.59062243825054));
#8363=CARTESIAN_POINT('Ctrl Pts',(-8.37303350223909,2.99748056064557,1.59062243825054));
#8364=CARTESIAN_POINT('Ctrl Pts',(-8.37303350223909,2.99748056064557,-2.37492204981212E-15));
#8365=CARTESIAN_POINT('Ctrl Pts',(-8.37303350223908,2.99748056064557,-1.59062243825055));
#8366=CARTESIAN_POINT('Ctrl Pts',(-7.57772228311383,4.3750000000001,-1.59062243825055));
#8367=CARTESIAN_POINT('Ctrl Pts',(-6.78241106398857,5.75251943935462,-1.59062243825054));
#8368=CARTESIAN_POINT('Ctrl Pts',(-6.78241106398857,5.75251943935462,-1.54476000561847E-16));
#8369=CARTESIAN_POINT('Ctrl Pts',(-6.78241106398857,5.75251943935462,1.59062243825054));
#8370=CARTESIAN_POINT('Ctrl Pts',(-7.57772228311383,4.3750000000001,1.59062243825054));
#8371=CARTESIAN_POINT('Ctrl Pts',(-7.14470958122158,4.12500000000008,1.77871997289448));
#8372=CARTESIAN_POINT('Ctrl Pts',(-8.0340695676688,2.58458331725469,1.77871997289448));
#8373=CARTESIAN_POINT('Ctrl Pts',(-8.0340695676688,2.58458331725469,-1.77809156287621E-15));
#8374=CARTESIAN_POINT('Ctrl Pts',(-8.03406956766879,2.58458331725469,-1.77871997289448));
#8375=CARTESIAN_POINT('Ctrl Pts',(-7.14470958122157,4.12500000000008,-1.77871997289448));
#8376=CARTESIAN_POINT('Ctrl Pts',(-6.25534959477435,5.66541668274548,-1.77871997289448));
#8377=CARTESIAN_POINT('Ctrl Pts',(-6.25534959477435,5.66541668274548,4.42354486374065E-16));
#8378=CARTESIAN_POINT('Ctrl Pts',(-6.25534959477435,5.66541668274548,1.77871997289448));
#8379=CARTESIAN_POINT('Ctrl Pts',(-7.14470958122158,4.12500000000008,1.77871997289448));
#8380=CARTESIAN_POINT('Ctrl Pts',(-6.71169687932932,3.87500000000007,1.59062243825054));
#8381=CARTESIAN_POINT('Ctrl Pts',(-7.50700809845458,2.49748056064554,1.59062243825054));
#8382=CARTESIAN_POINT('Ctrl Pts',(-7.50700809845458,2.49748056064554,-1.18126107594029E-15));
#8383=CARTESIAN_POINT('Ctrl Pts',(-7.50700809845457,2.49748056064554,-1.59062243825054));
#8384=CARTESIAN_POINT('Ctrl Pts',(-6.71169687932932,3.87500000000007,-1.59062243825054));
#8385=CARTESIAN_POINT('Ctrl Pts',(-5.91638566020406,5.25251943935459,-1.59062243825054));
#8386=CARTESIAN_POINT('Ctrl Pts',(-5.91638566020406,5.25251943935459,1.03918497330998E-15));
#8387=CARTESIAN_POINT('Ctrl Pts',(-5.91638566020406,5.25251943935459,1.59062243825054));
#8388=CARTESIAN_POINT('Ctrl Pts',(-6.71169687932932,3.87500000000007,1.59062243825054));
#8389=CARTESIAN_POINT('',(-6.71169687932935,3.87500000000008,1.59062243825056));
#8390=CARTESIAN_POINT('Origin',(-6.71169687932935,3.87500000000008,7.11825952004385E-16));
#8391=CARTESIAN_POINT('',(-7.57772228311379,4.37500000000009,1.59062243825056));
#8392=CARTESIAN_POINT('Origin',(-7.14470958122157,4.12500000000008,0.261524741817234));
#8393=CARTESIAN_POINT('Origin',(-7.57772228311379,4.37500000000009,8.03674461940435E-16));
#8394=CARTESIAN_POINT('Origin',(-7.14470958122157,4.12500000000008,-4.77168087270366E-15));
#8395=CARTESIAN_POINT('',(-7.89213313939235,2.83042442247442,-4.68014788589155E-15));
#8396=CARTESIAN_POINT('',(-6.3972860230508,5.41957557752574,-4.68014788589155E-15));
#8397=CARTESIAN_POINT('Origin',(-7.14470958122157,4.12500000000008,-4.77168087270366E-15));
#8398=CARTESIAN_POINT('',(-6.71169687932935,3.87500000000008,-1.40874692590067));
#8399=CARTESIAN_POINT('Origin',(-6.71169687932935,3.87500000000008,7.11825952004385E-16));
#8400=CARTESIAN_POINT('',(-7.57772228311379,4.37500000000009,-1.40874692590067));
#8401=CARTESIAN_POINT('Origin',(-7.57772228311379,4.37500000000009,8.03674461940435E-16));
#8402=CARTESIAN_POINT('Origin',(-7.57772228311379,4.37500000000009,-1.40874692590067));
#8403=CARTESIAN_POINT('Origin',(-6.71169687932935,3.87500000000008,-1.59062243825056));
#8404=CARTESIAN_POINT('Ctrl Pts',(-4.3749999999999,7.5777222831139,1.59062243825056));
#8405=CARTESIAN_POINT('Ctrl Pts',(-5.75251943935444,6.78241106398865,1.59062243825055));
#8406=CARTESIAN_POINT('Ctrl Pts',(-5.75251943935444,6.78241106398865,1.08090394793333E-15));
#8407=CARTESIAN_POINT('Ctrl Pts',(-5.75251943935444,6.78241106398866,-1.59062243825055));
#8408=CARTESIAN_POINT('Ctrl Pts',(-4.3749999999999,7.5777222831139,-1.59062243825055));
#8409=CARTESIAN_POINT('Ctrl Pts',(-2.99748056064537,8.37303350223915,-1.59062243825055));
#8410=CARTESIAN_POINT('Ctrl Pts',(-2.99748056064537,8.37303350223915,5.5217960464338E-15));
#8411=CARTESIAN_POINT('Ctrl Pts',(-2.99748056064537,8.37303350223915,1.59062243825056));
#8412=CARTESIAN_POINT('Ctrl Pts',(-4.3749999999999,7.5777222831139,1.59062243825056));
#8413=CARTESIAN_POINT('Ctrl Pts',(-4.12499999999991,7.14470958122166,1.77871997289447));
#8414=CARTESIAN_POINT('Ctrl Pts',(-5.6654166827453,6.25534959477446,1.77871997289446));
#8415=CARTESIAN_POINT('Ctrl Pts',(-5.6654166827453,6.25534959477447,-1.12757025938426E-16));
#8416=CARTESIAN_POINT('Ctrl Pts',(-5.6654166827453,6.25534959477447,-1.77871997289446));
#8417=CARTESIAN_POINT('Ctrl Pts',(-4.12499999999991,7.14470958122167,-1.77871997289446));
#8418=CARTESIAN_POINT('Ctrl Pts',(-2.58458331725452,8.03406956766888,-1.77871997289446));
#8419=CARTESIAN_POINT('Ctrl Pts',(-2.58458331725452,8.03406956766887,4.32813507256205E-15));
#8420=CARTESIAN_POINT('Ctrl Pts',(-2.58458331725452,8.03406956766887,1.77871997289447));
#8421=CARTESIAN_POINT('Ctrl Pts',(-4.12499999999991,7.14470958122166,1.77871997289447));
#8422=CARTESIAN_POINT('Ctrl Pts',(-3.87499999999991,6.71169687932943,1.59062243825055));
#8423=CARTESIAN_POINT('Ctrl Pts',(-5.25251943935445,5.91638566020418,1.59062243825055));
#8424=CARTESIAN_POINT('Ctrl Pts',(-5.25251943935445,5.91638566020419,-8.25677328214282E-16));
#8425=CARTESIAN_POINT('Ctrl Pts',(-5.25251943935445,5.91638566020419,-1.59062243825055));
#8426=CARTESIAN_POINT('Ctrl Pts',(-3.87499999999991,6.71169687932944,-1.59062243825055));
#8427=CARTESIAN_POINT('Ctrl Pts',(-2.49748056064538,7.50700809845469,-1.59062243825055));
#8428=CARTESIAN_POINT('Ctrl Pts',(-2.49748056064537,7.50700809845469,2.6537334270944E-15));
#8429=CARTESIAN_POINT('Ctrl Pts',(-2.49748056064537,7.50700809845468,1.59062243825055));
#8430=CARTESIAN_POINT('Ctrl Pts',(-3.87499999999991,6.71169687932943,1.59062243825055));
#8431=CARTESIAN_POINT('',(-3.87499999999991,6.71169687932945,1.59062243825056));
#8432=CARTESIAN_POINT('Origin',(-3.87499999999991,6.71169687932945,1.90733188991085E-16));
#8433=CARTESIAN_POINT('',(-4.3749999999999,7.57772228311389,1.59062243825056));
#8434=CARTESIAN_POINT('Origin',(-4.12499999999991,7.14470958122167,0.26152474181723));
#8435=CARTESIAN_POINT('Origin',(-4.3749999999999,7.57772228311389,2.15343923054451E-16));
#8436=CARTESIAN_POINT('Origin',(-4.12499999999991,7.14470958122167,-5.32639252365331E-15));
#8437=CARTESIAN_POINT('',(-5.41957557752559,6.39728602305093,-5.2348595368412E-15));
#8438=CARTESIAN_POINT('',(-2.83042442247423,7.89213313939241,-5.2348595368412E-15));
#8439=CARTESIAN_POINT('Origin',(-4.12499999999991,7.14470958122167,-5.32639252365331E-15));
#8440=CARTESIAN_POINT('',(-3.87499999999991,6.71169687932945,-1.40874692590067));
#8441=CARTESIAN_POINT('Origin',(-3.87499999999991,6.71169687932945,1.90733188991085E-16));
#8442=CARTESIAN_POINT('',(-4.3749999999999,7.5777222831139,-1.40874692590067));
#8443=CARTESIAN_POINT('Origin',(-4.3749999999999,7.57772228311389,2.15343923054451E-16));
#8444=CARTESIAN_POINT('Origin',(-4.3749999999999,7.57772228311389,-1.40874692590067));
#8445=CARTESIAN_POINT('Origin',(-3.87499999999991,6.71169687932945,-1.59062243825056));
#8446=CARTESIAN_POINT('Origin',(-7.14470958122157,4.12500000000008,7.5775020697241E-16));
#8447=CARTESIAN_POINT('',(-7.89213313939235,2.83042442247441,9.95559882563082E-16));
#8448=CARTESIAN_POINT('',(-6.39728602305079,5.41957557752575,5.19940531381738E-16));
#8449=CARTESIAN_POINT('Origin',(-7.14470958122157,4.12500000000008,7.5775020697241E-16));
#8450=CARTESIAN_POINT('Origin',(-4.12499999999991,7.14470958122167,2.03038556022768E-16));
#8451=CARTESIAN_POINT('',(-5.4195755775256,6.39728602305092,3.40338036240938E-16));
#8452=CARTESIAN_POINT('',(-2.83042442247422,7.89213313939242,6.5739075804598E-17));
#8453=CARTESIAN_POINT('Origin',(-4.12499999999991,7.14470958122167,2.03038556022768E-16));
#8454=CARTESIAN_POINT('Origin',(0.,5.1026949964479E-18,-2.47222222222222));
#8455=CARTESIAN_POINT('',(-9.09640428033339E-16,-7.42777777777777,-2.5));
#8456=CARTESIAN_POINT('Origin',(0.,6.13137853388905E-31,-2.5));
#8457=CARTESIAN_POINT('',(9.0623863136904E-16,-7.39999999999999,-2.47222222222222));
#8458=CARTESIAN_POINT('Origin',(9.09640428033339E-16,-7.42777777777777,
-2.47222222222222));
#8459=CARTESIAN_POINT('',(9.06238631369041E-16,7.39999999999999,-2.47222222222222));
#8460=CARTESIAN_POINT('Origin',(0.,5.1026949964479E-18,-2.47222222222222));
#8461=CARTESIAN_POINT('Origin',(0.,5.1026949964479E-18,-2.47222222222222));
#8462=CARTESIAN_POINT('Origin',(0.,5.1026949964479E-18,-2.47222222222222));
#8463=CARTESIAN_POINT('',(1.11442858722409E-15,9.1,-2.47222222222222));
#8464=CARTESIAN_POINT('',(1.11442858722409E-15,-9.1,-2.47222222222222));
#8465=CARTESIAN_POINT('Origin',(0.,5.10269499644792E-18,-2.47222222222222));
#8466=CARTESIAN_POINT('',(-1.11102679055979E-15,-9.07222222222223,-2.5));
#8467=CARTESIAN_POINT('Origin',(1.11102679055979E-15,-9.07222222222223,
-2.47222222222222));
#8468=CARTESIAN_POINT('Origin',(0.,6.13137853388905E-31,-2.5));
#8469=CARTESIAN_POINT('Origin',(0.,5.10269499644792E-18,-2.47222222222222));
#8470=CARTESIAN_POINT('Origin',(0.,0.,-2.5));
#8471=CARTESIAN_POINT('',(1.1236134382177E-15,-9.1,-2.31481481481481));
#8472=CARTESIAN_POINT('',(-1.11442858722409E-15,9.1,-2.31481481481481));
#8473=CARTESIAN_POINT('Origin',(0.,3.40179666429828E-17,-2.31481481481481));
#8474=CARTESIAN_POINT('Origin',(0.,3.40179666429828E-17,-2.31481481481481));
#8475=CARTESIAN_POINT('',(-1.11442858722409E-15,9.1,-2.5));
#8476=CARTESIAN_POINT('Origin',(0.,5.10269499644737E-17,-2.22222222222222));
#8477=CARTESIAN_POINT('',(-1.1327982892113E-15,-9.25000000000001,-2.22222222222222));
#8478=CARTESIAN_POINT('Origin',(0.,5.10269499644737E-17,-2.22222222222222));
#8479=CARTESIAN_POINT('',(1.1327982892113E-15,-9.25000000000001,-2.22222222222222));
#8480=CARTESIAN_POINT('Origin',(0.,3.40179666429827E-17,-2.31481481481481));
#8481=CARTESIAN_POINT('',(-8.8786892938183E-16,7.24999999999999,-2.22222222222222));
#8482=CARTESIAN_POINT('Origin',(0.,5.10269499644738E-17,-2.22222222222222));
#8483=CARTESIAN_POINT('',(-9.06238631369041E-16,7.39999999999999,-2.31481481481481));
#8484=CARTESIAN_POINT('',(9.0623863136904E-16,7.39999999999999,-2.31481481481481));
#8485=CARTESIAN_POINT('Origin',(0.,3.40179666429827E-17,-2.31481481481481));
#8486=CARTESIAN_POINT('Origin',(0.,0.,-2.5));
#8487=CARTESIAN_POINT('',(-9.0623863136904E-16,7.39999999999999,-2.5));
#8488=CARTESIAN_POINT('Origin',(0.,9.1,-2.5));
#8489=CARTESIAN_POINT('Origin',(0.,9.25000000000001,-2.22222222222222));
#8490=CARTESIAN_POINT('Origin',(0.,9.13382404364069E-16,2.47222222222223));
#8491=CARTESIAN_POINT('',(-1.11442858722409E-15,9.1,2.47222222222223));
#8492=CARTESIAN_POINT('Origin',(0.,9.13382404364069E-16,2.47222222222223));
#8493=CARTESIAN_POINT('',(-1.11102679055979E-15,9.07222222222223,2.50000000000001));
#8494=CARTESIAN_POINT('Origin',(1.11102679055979E-15,9.07222222222222,2.47222222222223));
#8495=CARTESIAN_POINT('Origin',(0.,9.18485099360517E-16,2.50000000000001));
#8496=CARTESIAN_POINT('Origin',(0.,9.13382404364069E-16,2.47222222222223));
#8497=CARTESIAN_POINT('',(-9.09640428033339E-16,7.42777777777777,2.50000000000001));
#8498=CARTESIAN_POINT('Origin',(0.,9.18485099360517E-16,2.50000000000001));
#8499=CARTESIAN_POINT('',(-9.06238631369041E-16,7.39999999999999,2.47222222222223));
#8500=CARTESIAN_POINT('Origin',(9.09640428033339E-16,7.42777777777777,2.47222222222223));
#8501=CARTESIAN_POINT('Origin',(0.,9.13382404364069E-16,2.47222222222223));
#8502=CARTESIAN_POINT('Origin',(0.,0.,-2.5));
#8503=CARTESIAN_POINT('',(9.06238631369041E-16,-7.39999999999999,2.31481481481482));
#8504=CARTESIAN_POINT('',(-9.0623863136904E-16,7.39999999999999,2.31481481481482));
#8505=CARTESIAN_POINT('Origin',(0.,8.84467132717534E-16,2.31481481481482));
#8506=CARTESIAN_POINT('Origin',(0.,8.84467132717534E-16,2.31481481481482));
#8507=CARTESIAN_POINT('',(-9.0623863136904E-16,7.39999999999999,-2.5));
#8508=CARTESIAN_POINT('Origin',(0.,8.67458149396043E-16,2.22222222222223));
#8509=CARTESIAN_POINT('',(-8.8786892938183E-16,-7.24999999999999,2.22222222222223));
#8510=CARTESIAN_POINT('Origin',(0.,8.67458149396043E-16,2.22222222222223));
#8511=CARTESIAN_POINT('',(8.8786892938183E-16,-7.24999999999999,2.22222222222223));
#8512=CARTESIAN_POINT('Origin',(0.,8.84467132717534E-16,2.31481481481482));
#8513=CARTESIAN_POINT('',(-1.1327982892113E-15,9.25000000000001,2.22222222222223));
#8514=CARTESIAN_POINT('Origin',(0.,8.67458149396044E-16,2.22222222222223));
#8515=CARTESIAN_POINT('',(-1.11442858722409E-15,9.1,2.31481481481482));
#8516=CARTESIAN_POINT('',(1.11442858722409E-15,9.1,2.31481481481482));
#8517=CARTESIAN_POINT('Origin',(0.,8.84467132717534E-16,2.31481481481482));
#8518=CARTESIAN_POINT('Origin',(0.,0.,-2.5));
#8519=CARTESIAN_POINT('',(-1.11442858722409E-15,9.1,-2.5));
#8520=CARTESIAN_POINT('Origin',(0.,7.24999999999999,2.22222222222223));
#8521=CARTESIAN_POINT('Origin',(0.,9.1,2.50000000000001));
#9478=UNCERTAINTY_MEASURE_WITH_UNIT(LENGTH_MEASURE(0.01),#9497,
'DISTANCE_ACCURACY_VALUE',
'Maximum model space distance between geometric entities at asserted c
onnectivities');
#9485=UNCERTAINTY_MEASURE_WITH_UNIT(LENGTH_MEASURE(0.01),#9497,
'DISTANCE_ACCURACY_VALUE',
'Maximum model space distance between geometric entities at asserted c
onnectivities');
#9489=(
GEOMETRIC_REPRESENTATION_CONTEXT(3)
GLOBAL_UNCERTAINTY_ASSIGNED_CONTEXT((#9478))
GLOBAL_UNIT_ASSIGNED_CONTEXT((#9497,#9499,#9500))
REPRESENTATION_CONTEXT('','3D')
);
#9496=(
GEOMETRIC_REPRESENTATION_CONTEXT(3)
GLOBAL_UNCERTAINTY_ASSIGNED_CONTEXT((#9485))
GLOBAL_UNIT_ASSIGNED_CONTEXT((#9497,#9499,#9500))
REPRESENTATION_CONTEXT('','3D')
);
#9497=(
LENGTH_UNIT()
NAMED_UNIT(*)
SI_UNIT(.MILLI.,.METRE.)
);
#9499=(
NAMED_UNIT(*)
PLANE_ANGLE_UNIT()
SI_UNIT($,.RADIAN.)
);
#9500=(
NAMED_UNIT(*)
SI_UNIT($,.STERADIAN.)
SOLID_ANGLE_UNIT()
);
#9504=SHAPE_DEFINITION_REPRESENTATION(#9514,#9541);
#9514=PRODUCT_DEFINITION_SHAPE('',$,#9552);
#9541=SHAPE_REPRESENTATION('',(#5298),#9489);
#9548=PRODUCT_DEFINITION_CONTEXT('part definition',#9580,'design');
#9552=PRODUCT_DEFINITION('Ball Bearing - Small','Ball Bearing - Small',
#9562,#9548);
#9562=PRODUCT_DEFINITION_FORMATION('',$,#9585);
#9580=APPLICATION_CONTEXT(
'Core Data for Automotive Mechanical Design Process');
#9581=PRODUCT_CONTEXT('part definition',#9580,'mechanical');
#9585=PRODUCT('Ball Bearing - Small','Ball Bearing - Small',$,(#9581));
#9594=PRESENTATION_STYLE_ASSIGNMENT((#9597));
#9597=SURFACE_STYLE_USAGE(.BOTH.,#9600);
#9600=SURFACE_SIDE_STYLE('',(#9603));
#9603=SURFACE_STYLE_FILL_AREA(#9606);
#9606=FILL_AREA_STYLE('Opaque(160,160,160)',(#9609));
#9609=FILL_AREA_STYLE_COLOUR('Opaque(160,160,160)',#9612);
#9612=COLOUR_RGB('Opaque(160,160,160)', 0.40784314, 0.44705882, 0.49803922);
ENDSEC;
END-ISO-10303-21;
